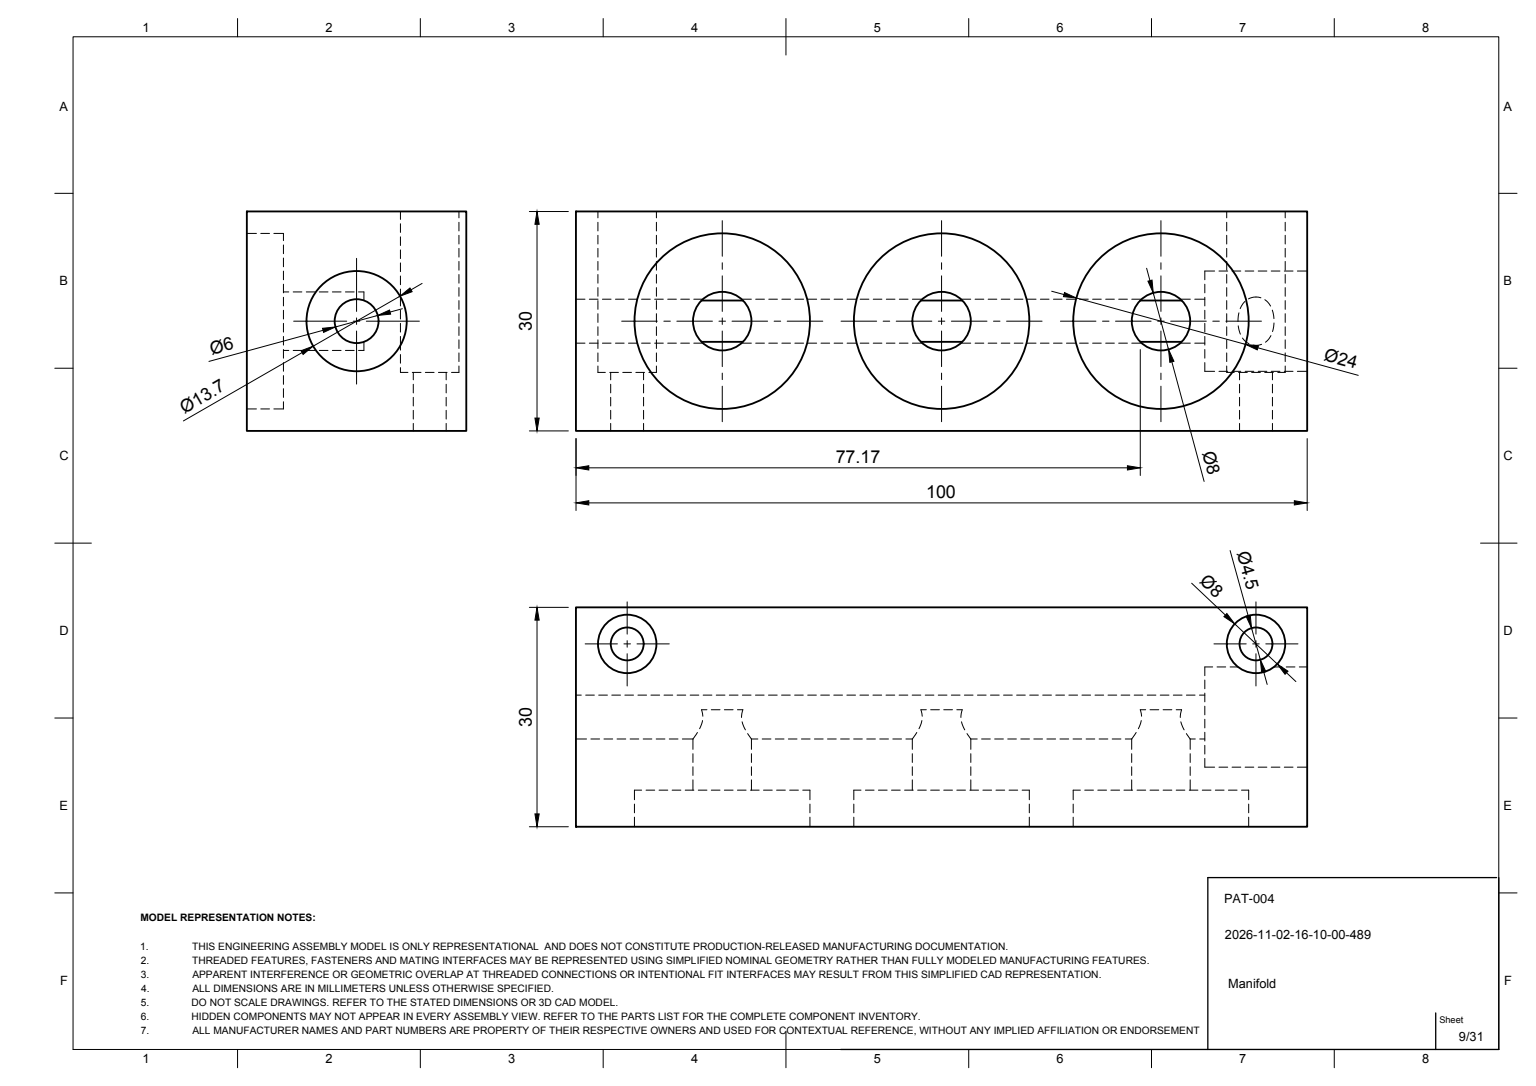
ISO-10303-21;
HEADER;
/* Generated by software containing ST-Developer
 * from STEP Tools, Inc. (www.steptools.com) 
 */

FILE_DESCRIPTION(
/* description */ ('Air blow-off nozzle station'),
/* implementation_level */ '2;1');

FILE_NAME(
/* name */ 'Manifold.step',
/* time_stamp */ '2026-10-27T10:53:54-07:00',
/* author */ (''),
/* organization */ (''),
/* preprocessor_version */ 'ST-DEVELOPER v20.2',
/* originating_system */ 'Autodesk Translation Framework v15.17.0.0',
/* authorisation */ '');

FILE_SCHEMA (('AUTOMOTIVE_DESIGN { 1 0 10303 214 3 1 1 }'));
ENDSEC;

DATA;
#10=MECHANICAL_DESIGN_GEOMETRIC_PRESENTATION_REPRESENTATION('',(#241),#7897);
#171=B_SPLINE_CURVE_WITH_KNOTS('',3,(#6538,#6539,#6540,#6541,#6542,#6543,
#6544,#6545,#6546,#6547,#6548,#6549),.UNSPECIFIED.,.F.,.F.,(4,2,2,2,2,4),
(-0.956775615070493,-0.896341583425285,-0.835907551780076,-0.715039488489658,
-0.596713648012452,-0.478387807535247),.UNSPECIFIED.);
#172=B_SPLINE_CURVE_WITH_KNOTS('',3,(#6550,#6551,#6552,#6553,#6554,#6555),
 .UNSPECIFIED.,.F.,.F.,(4,2,4),(-1.05899336181655,-1.0172096467157,-0.956775615070493),
 .UNSPECIFIED.);
#173=B_SPLINE_CURVE_WITH_KNOTS('',3,(#6557,#6558,#6559,#6560,#6561,#6562),
 .UNSPECIFIED.,.F.,.F.,(4,2,4),(0.956775615070494,1.0172096467157,1.0589933625076),
 .UNSPECIFIED.);
#174=B_SPLINE_CURVE_WITH_KNOTS('',3,(#6564,#6565,#6566,#6567,#6568,#6569,
#6570,#6571,#6572,#6573,#6574,#6575,#6576,#6577,#6578,#6579,#6580,#6581,
#6582,#6583,#6584,#6585,#6586,#6587,#6588,#6589,#6590),.UNSPECIFIED.,.F.,
 .F.,(4,2,3,2,2,2,2,2,2,2,2,2,4),(-0.102217746746059,-0.0604340316452088,
0.,0.0604340316452089,0.120868063290418,0.241736126580836,0.360061967058041,
0.478387807535247,0.596713648012453,0.715039488489658,0.835907551780076,
0.896341583425285,0.956775615070494),.UNSPECIFIED.);
#175=B_SPLINE_CURVE_WITH_KNOTS('',3,(#6593,#6594,#6595,#6596,#6597,#6598,
#6599,#6600,#6601,#6602,#6603,#6604,#6605,#6606,#6607,#6608,#6609),
 .UNSPECIFIED.,.F.,.F.,(4,2,2,2,2,3,2,4),(-0.478387807535247,-0.360061967058041,
-0.241736126580835,-0.120868063290418,-0.0604340316452086,2.22044604925031E-16,
0.0604340316452088,0.102217747437109),.UNSPECIFIED.);
#176=B_SPLINE_CURVE_WITH_KNOTS('',3,(#6630,#6631,#6632,#6633,#6634,#6635,
#6636,#6637,#6638,#6639,#6640,#6641),.UNSPECIFIED.,.F.,.F.,(4,2,2,2,2,4),
(-0.956775615070493,-0.896341583425285,-0.835907551780076,-0.715039488489658,
-0.596713648012452,-0.478387807535247),.UNSPECIFIED.);
#177=B_SPLINE_CURVE_WITH_KNOTS('',3,(#6642,#6643,#6644,#6645,#6646,#6647),
 .UNSPECIFIED.,.F.,.F.,(4,2,4),(-1.05899336181655,-1.0172096467157,-0.956775615070493),
 .UNSPECIFIED.);
#178=B_SPLINE_CURVE_WITH_KNOTS('',3,(#6649,#6650,#6651,#6652,#6653,#6654),
 .UNSPECIFIED.,.F.,.F.,(4,2,4),(0.956775615070493,1.0172096467157,1.0589933625076),
 .UNSPECIFIED.);
#179=B_SPLINE_CURVE_WITH_KNOTS('',3,(#6656,#6657,#6658,#6659,#6660,#6661,
#6662,#6663,#6664,#6665,#6666,#6667,#6668,#6669,#6670,#6671,#6672,#6673,
#6674,#6675,#6676,#6677,#6678,#6679,#6680,#6681,#6682),.UNSPECIFIED.,.F.,
 .F.,(4,2,3,2,2,2,2,2,2,2,2,2,4),(-0.102217746746057,-0.0604340316452088,
0.,0.0604340316452089,0.120868063290418,0.241736126580835,0.360061967058041,
0.478387807535247,0.596713648012452,0.715039488489658,0.835907551780075,
0.896341583425284,0.956775615070493),.UNSPECIFIED.);
#180=B_SPLINE_CURVE_WITH_KNOTS('',3,(#6685,#6686,#6687,#6688,#6689,#6690,
#6691,#6692,#6693,#6694,#6695,#6696,#6697,#6698,#6699,#6700,#6701),
 .UNSPECIFIED.,.F.,.F.,(4,2,2,2,2,3,2,4),(-0.478387807535247,-0.360061967058041,
-0.241736126580836,-0.120868063290418,-0.060434031645209,0.,0.0604340316452088,
0.102217747437111),.UNSPECIFIED.);
#181=B_SPLINE_CURVE_WITH_KNOTS('',3,(#6722,#6723,#6724,#6725,#6726,#6727,
#6728,#6729,#6730,#6731,#6732,#6733),.UNSPECIFIED.,.F.,.F.,(4,2,2,2,2,4),
(-0.956775615070493,-0.896341583425285,-0.835907551780076,-0.715039488489658,
-0.596713648012452,-0.478387807535247),.UNSPECIFIED.);
#182=B_SPLINE_CURVE_WITH_KNOTS('',3,(#6734,#6735,#6736,#6737,#6738,#6739),
 .UNSPECIFIED.,.F.,.F.,(4,2,4),(-1.05899336181655,-1.0172096467157,-0.956775615070493),
 .UNSPECIFIED.);
#183=B_SPLINE_CURVE_WITH_KNOTS('',3,(#6741,#6742,#6743,#6744,#6745,#6746),
 .UNSPECIFIED.,.F.,.F.,(4,2,4),(0.956775615070494,1.0172096467157,1.0589933625076),
 .UNSPECIFIED.);
#184=B_SPLINE_CURVE_WITH_KNOTS('',3,(#6748,#6749,#6750,#6751,#6752,#6753,
#6754,#6755,#6756,#6757,#6758,#6759,#6760,#6761,#6762,#6763,#6764,#6765,
#6766,#6767,#6768,#6769,#6770,#6771,#6772,#6773,#6774),.UNSPECIFIED.,.F.,
 .F.,(4,2,3,2,2,2,2,2,2,2,2,2,4),(-0.102217746746057,-0.0604340316452088,
0.,0.0604340316452089,0.120868063290418,0.241736126580836,0.360061967058041,
0.478387807535247,0.596713648012453,0.715039488489658,0.835907551780076,
0.896341583425285,0.956775615070494),.UNSPECIFIED.);
#185=B_SPLINE_CURVE_WITH_KNOTS('',3,(#6777,#6778,#6779,#6780,#6781,#6782,
#6783,#6784,#6785,#6786,#6787,#6788,#6789,#6790,#6791,#6792,#6793),
 .UNSPECIFIED.,.F.,.F.,(4,2,2,2,2,3,2,4),(-0.478387807535247,-0.360061967058041,
-0.241736126580835,-0.120868063290418,-0.0604340316452086,2.22044604925031E-16,
0.0604340316452088,0.102217747437111),.UNSPECIFIED.);
#186=B_SPLINE_CURVE_WITH_KNOTS('',3,(#6810,#6811,#6812,#6813,#6814,#6815,
#6816,#6817,#6818,#6819,#6820,#6821,#6822,#6823,#6824,#6825,#6826,#6827,
#6828,#6829,#6830,#6831,#6832,#6833,#6834,#6835,#6836,#6837,#6838,#6839,
#6840,#6841,#6842,#6843,#6844,#6845,#6846,#6847,#6848,#6849,#6850,#6851),
 .UNSPECIFIED.,.T.,.F.,(4,2,2,2,2,2,2,2,2,2,2,2,2,2,2,2,2,2,2,2,4),(0.,
0.0876674059984988,0.175334811996998,0.268557118055512,0.358098480537522,
0.447639843019532,0.537181205501541,0.626722567983551,0.719944874042066,
0.807612280040565,0.895279686039063,0.982947092037562,1.07061449803606,
1.16383680409458,1.25337816657659,1.3429195290586,1.43246089154061,1.52200225402261,
1.61522456008113,1.70289196607963,1.79055937207813),.UNSPECIFIED.);
#191=SHAPE_REPRESENTATION_RELATIONSHIP('SRR','None',#8005,#216);
#216=ADVANCED_BREP_SHAPE_REPRESENTATION('',(#266),#7872);
#241=STYLED_ITEM('',(#8234),#266);
#266=MANIFOLD_SOLID_BREP('Body1',#4290);
#293=FACE_BOUND('',#837,.T.);
#294=FACE_BOUND('',#843,.T.);
#295=FACE_BOUND('',#849,.T.);
#296=FACE_BOUND('',#851,.T.);
#297=FACE_BOUND('',#853,.T.);
#298=FACE_BOUND('',#857,.T.);
#299=FACE_BOUND('',#859,.T.);
#300=FACE_BOUND('',#861,.T.);
#301=FACE_BOUND('',#866,.T.);
#302=FACE_BOUND('',#868,.T.);
#303=FACE_BOUND('',#869,.T.);
#304=FACE_BOUND('',#870,.T.);
#305=FACE_BOUND('',#872,.T.);
#306=FACE_BOUND('',#874,.T.);
#307=FACE_BOUND('',#875,.T.);
#308=FACE_BOUND('',#877,.T.);
#309=FACE_BOUND('',#878,.T.);
#395=PLANE('',#4632);
#396=PLANE('',#4637);
#397=PLANE('',#4641);
#398=PLANE('',#4642);
#399=PLANE('',#4647);
#400=PLANE('',#4651);
#401=PLANE('',#4652);
#402=PLANE('',#4657);
#403=PLANE('',#4661);
#404=PLANE('',#4665);
#405=PLANE('',#4672);
#406=PLANE('',#4677);
#407=PLANE('',#4683);
#408=PLANE('',#4684);
#409=PLANE('',#4685);
#410=PLANE('',#4686);
#411=PLANE('',#4687);
#412=PLANE('',#4688);
#568=FACE_OUTER_BOUND('',#832,.T.);
#569=FACE_OUTER_BOUND('',#833,.T.);
#570=FACE_OUTER_BOUND('',#834,.T.);
#571=FACE_OUTER_BOUND('',#835,.T.);
#572=FACE_OUTER_BOUND('',#836,.T.);
#573=FACE_OUTER_BOUND('',#838,.T.);
#574=FACE_OUTER_BOUND('',#839,.T.);
#575=FACE_OUTER_BOUND('',#840,.T.);
#576=FACE_OUTER_BOUND('',#841,.T.);
#577=FACE_OUTER_BOUND('',#842,.T.);
#578=FACE_OUTER_BOUND('',#844,.T.);
#579=FACE_OUTER_BOUND('',#845,.T.);
#580=FACE_OUTER_BOUND('',#846,.T.);
#581=FACE_OUTER_BOUND('',#847,.T.);
#582=FACE_OUTER_BOUND('',#848,.T.);
#583=FACE_OUTER_BOUND('',#850,.T.);
#584=FACE_OUTER_BOUND('',#852,.T.);
#585=FACE_OUTER_BOUND('',#854,.T.);
#586=FACE_OUTER_BOUND('',#855,.T.);
#587=FACE_OUTER_BOUND('',#856,.T.);
#588=FACE_OUTER_BOUND('',#858,.T.);
#589=FACE_OUTER_BOUND('',#860,.T.);
#590=FACE_OUTER_BOUND('',#862,.T.);
#591=FACE_OUTER_BOUND('',#863,.T.);
#592=FACE_OUTER_BOUND('',#864,.T.);
#593=FACE_OUTER_BOUND('',#865,.T.);
#594=FACE_OUTER_BOUND('',#867,.T.);
#595=FACE_OUTER_BOUND('',#871,.T.);
#596=FACE_OUTER_BOUND('',#873,.T.);
#597=FACE_OUTER_BOUND('',#876,.T.);
#832=EDGE_LOOP('',(#3017,#3018));
#833=EDGE_LOOP('',(#3019,#3020,#3021,#3022,#3023,#3024,#3025,#3026,#3027,
#3028));
#834=EDGE_LOOP('',(#3029,#3030));
#835=EDGE_LOOP('',(#3031,#3032,#3033,#3034));
#836=EDGE_LOOP('',(#3035));
#837=EDGE_LOOP('',(#3036));
#838=EDGE_LOOP('',(#3037,#3038));
#839=EDGE_LOOP('',(#3039,#3040,#3041,#3042,#3043,#3044,#3045,#3046,#3047,
#3048));
#840=EDGE_LOOP('',(#3049,#3050));
#841=EDGE_LOOP('',(#3051,#3052,#3053,#3054));
#842=EDGE_LOOP('',(#3055));
#843=EDGE_LOOP('',(#3056));
#844=EDGE_LOOP('',(#3057,#3058));
#845=EDGE_LOOP('',(#3059,#3060,#3061,#3062,#3063,#3064,#3065,#3066,#3067,
#3068));
#846=EDGE_LOOP('',(#3069,#3070));
#847=EDGE_LOOP('',(#3071,#3072,#3073,#3074));
#848=EDGE_LOOP('',(#3075));
#849=EDGE_LOOP('',(#3076));
#850=EDGE_LOOP('',(#3077,#3078,#3079,#3080));
#851=EDGE_LOOP('',(#3081));
#852=EDGE_LOOP('',(#3082));
#853=EDGE_LOOP('',(#3083));
#854=EDGE_LOOP('',(#3084,#3085,#3086,#3087,#3088,#3089,#3090,#3091,#3092,
#3093,#3094,#3095,#3096,#3097,#3098,#3099,#3100,#3101,#3102,#3103,#3104,
#3105,#3106,#3107,#3108,#3109,#3110,#3111,#3112,#3113,#3114));
#855=EDGE_LOOP('',(#3115,#3116,#3117,#3118));
#856=EDGE_LOOP('',(#3119));
#857=EDGE_LOOP('',(#3120));
#858=EDGE_LOOP('',(#3121,#3122,#3123,#3124));
#859=EDGE_LOOP('',(#3125));
#860=EDGE_LOOP('',(#3126));
#861=EDGE_LOOP('',(#3127));
#862=EDGE_LOOP('',(#3128,#3129,#3130,#3131));
#863=EDGE_LOOP('',(#3132,#3133,#3134,#3135));
#864=EDGE_LOOP('',(#3136,#3137,#3138,#3139));
#865=EDGE_LOOP('',(#3140,#3141,#3142,#3143));
#866=EDGE_LOOP('',(#3144));
#867=EDGE_LOOP('',(#3145,#3146,#3147,#3148));
#868=EDGE_LOOP('',(#3149));
#869=EDGE_LOOP('',(#3150));
#870=EDGE_LOOP('',(#3151));
#871=EDGE_LOOP('',(#3152,#3153,#3154,#3155));
#872=EDGE_LOOP('',(#3156));
#873=EDGE_LOOP('',(#3157,#3158,#3159,#3160));
#874=EDGE_LOOP('',(#3161));
#875=EDGE_LOOP('',(#3162));
#876=EDGE_LOOP('',(#3163,#3164,#3165,#3166));
#877=EDGE_LOOP('',(#3167));
#878=EDGE_LOOP('',(#3168));
#1190=LINE('',#6530,#1544);
#1191=LINE('',#6536,#1545);
#1192=LINE('',#6611,#1546);
#1193=LINE('',#6616,#1547);
#1194=LINE('',#6622,#1548);
#1195=LINE('',#6628,#1549);
#1196=LINE('',#6703,#1550);
#1197=LINE('',#6708,#1551);
#1198=LINE('',#6714,#1552);
#1199=LINE('',#6720,#1553);
#1200=LINE('',#6795,#1554);
#1201=LINE('',#6800,#1555);
#1202=LINE('',#6807,#1556);
#1203=LINE('',#6858,#1557);
#1204=LINE('',#6859,#1558);
#1205=LINE('',#6860,#1559);
#1206=LINE('',#6861,#1560);
#1207=LINE('',#6866,#1561);
#1208=LINE('',#6875,#1562);
#1209=LINE('',#6883,#1563);
#1210=LINE('',#6887,#1564);
#1211=LINE('',#6891,#1565);
#1212=LINE('',#6893,#1566);
#1213=LINE('',#6895,#1567);
#1214=LINE('',#6896,#1568);
#1215=LINE('',#6899,#1569);
#1216=LINE('',#6901,#1570);
#1217=LINE('',#6902,#1571);
#1218=LINE('',#6905,#1572);
#1219=LINE('',#6907,#1573);
#1220=LINE('',#6908,#1574);
#1221=LINE('',#6910,#1575);
#1222=LINE('',#6911,#1576);
#1544=VECTOR('',#5212,1.);
#1545=VECTOR('',#5219,0.4);
#1546=VECTOR('',#5224,1.);
#1547=VECTOR('',#5229,1.2);
#1548=VECTOR('',#5236,1.);
#1549=VECTOR('',#5243,0.4);
#1550=VECTOR('',#5248,1.);
#1551=VECTOR('',#5253,1.2);
#1552=VECTOR('',#5260,1.);
#1553=VECTOR('',#5267,0.4);
#1554=VECTOR('',#5272,1.);
#1555=VECTOR('',#5277,1.2);
#1556=VECTOR('',#5286,0.684999999999999);
#1557=VECTOR('',#5297,0.300000000000001);
#1558=VECTOR('',#5298,0.300000000000001);
#1559=VECTOR('',#5299,0.300000000000001);
#1560=VECTOR('',#5300,0.300000000000001);
#1561=VECTOR('',#5305,0.4);
#1562=VECTOR('',#5316,0.4);
#1563=VECTOR('',#5327,0.225);
#1564=VECTOR('',#5332,0.225);
#1565=VECTOR('',#5335,1.);
#1566=VECTOR('',#5336,1.);
#1567=VECTOR('',#5337,1.);
#1568=VECTOR('',#5338,1.);
#1569=VECTOR('',#5341,1.);
#1570=VECTOR('',#5342,1.);
#1571=VECTOR('',#5343,1.);
#1572=VECTOR('',#5346,1.);
#1573=VECTOR('',#5347,1.);
#1574=VECTOR('',#5348,1.);
#1575=VECTOR('',#5351,1.);
#1576=VECTOR('',#5352,1.);
#1854=CIRCLE('',#4633,0.4);
#1855=CIRCLE('',#4635,0.4);
#1856=CIRCLE('',#4636,0.4);
#1857=CIRCLE('',#4639,1.2);
#1858=CIRCLE('',#4640,1.2);
#1859=CIRCLE('',#4643,0.4);
#1860=CIRCLE('',#4645,0.4);
#1861=CIRCLE('',#4646,0.4);
#1862=CIRCLE('',#4649,1.2);
#1863=CIRCLE('',#4650,1.2);
#1864=CIRCLE('',#4653,0.4);
#1865=CIRCLE('',#4655,0.4);
#1866=CIRCLE('',#4656,0.4);
#1867=CIRCLE('',#4659,1.2);
#1868=CIRCLE('',#4660,1.2);
#1869=CIRCLE('',#4663,0.684999999999999);
#1870=CIRCLE('',#4664,0.684999999999999);
#1871=CIRCLE('',#4666,0.300000000000001);
#1872=CIRCLE('',#4668,0.300000000000001);
#1873=CIRCLE('',#4670,0.4);
#1874=CIRCLE('',#4671,0.4);
#1875=CIRCLE('',#4673,0.225);
#1876=CIRCLE('',#4675,0.4);
#1877=CIRCLE('',#4676,0.4);
#1878=CIRCLE('',#4678,0.225);
#1879=CIRCLE('',#4680,0.225);
#1880=CIRCLE('',#4682,0.225);
#2047=VERTEX_POINT('',#6528);
#2048=VERTEX_POINT('',#6529);
#2049=VERTEX_POINT('',#6533);
#2050=VERTEX_POINT('',#6535);
#2051=VERTEX_POINT('',#6537);
#2052=VERTEX_POINT('',#6556);
#2053=VERTEX_POINT('',#6563);
#2054=VERTEX_POINT('',#6591);
#2055=VERTEX_POINT('',#6613);
#2056=VERTEX_POINT('',#6615);
#2057=VERTEX_POINT('',#6620);
#2058=VERTEX_POINT('',#6621);
#2059=VERTEX_POINT('',#6625);
#2060=VERTEX_POINT('',#6627);
#2061=VERTEX_POINT('',#6629);
#2062=VERTEX_POINT('',#6648);
#2063=VERTEX_POINT('',#6655);
#2064=VERTEX_POINT('',#6683);
#2065=VERTEX_POINT('',#6705);
#2066=VERTEX_POINT('',#6707);
#2067=VERTEX_POINT('',#6712);
#2068=VERTEX_POINT('',#6713);
#2069=VERTEX_POINT('',#6717);
#2070=VERTEX_POINT('',#6719);
#2071=VERTEX_POINT('',#6721);
#2072=VERTEX_POINT('',#6740);
#2073=VERTEX_POINT('',#6747);
#2074=VERTEX_POINT('',#6775);
#2075=VERTEX_POINT('',#6797);
#2076=VERTEX_POINT('',#6799);
#2077=VERTEX_POINT('',#6804);
#2078=VERTEX_POINT('',#6806);
#2079=VERTEX_POINT('',#6809);
#2080=VERTEX_POINT('',#6853);
#2081=VERTEX_POINT('',#6856);
#2082=VERTEX_POINT('',#6863);
#2083=VERTEX_POINT('',#6865);
#2084=VERTEX_POINT('',#6869);
#2085=VERTEX_POINT('',#6872);
#2086=VERTEX_POINT('',#6874);
#2087=VERTEX_POINT('',#6878);
#2088=VERTEX_POINT('',#6881);
#2089=VERTEX_POINT('',#6885);
#2090=VERTEX_POINT('',#6889);
#2091=VERTEX_POINT('',#6890);
#2092=VERTEX_POINT('',#6892);
#2093=VERTEX_POINT('',#6894);
#2094=VERTEX_POINT('',#6898);
#2095=VERTEX_POINT('',#6900);
#2096=VERTEX_POINT('',#6904);
#2097=VERTEX_POINT('',#6906);
#2426=EDGE_CURVE('',#2047,#2048,#1190,.T.);
#2427=EDGE_CURVE('',#2048,#2047,#1854,.T.);
#2428=EDGE_CURVE('',#2049,#2049,#1855,.T.);
#2429=EDGE_CURVE('',#2049,#2050,#1191,.T.);
#2430=EDGE_CURVE('',#2051,#2050,#171,.T.);
#2431=EDGE_CURVE('',#2048,#2051,#172,.T.);
#2432=EDGE_CURVE('',#2052,#2047,#173,.T.);
#2433=EDGE_CURVE('',#2053,#2052,#174,.T.);
#2434=EDGE_CURVE('',#2053,#2054,#1856,.T.);
#2435=EDGE_CURVE('',#2050,#2054,#175,.T.);
#2436=EDGE_CURVE('',#2054,#2053,#1192,.T.);
#2437=EDGE_CURVE('',#2055,#2055,#1857,.T.);
#2438=EDGE_CURVE('',#2055,#2056,#1193,.T.);
#2439=EDGE_CURVE('',#2056,#2056,#1858,.T.);
#2440=EDGE_CURVE('',#2057,#2058,#1194,.T.);
#2441=EDGE_CURVE('',#2058,#2057,#1859,.T.);
#2442=EDGE_CURVE('',#2059,#2059,#1860,.T.);
#2443=EDGE_CURVE('',#2059,#2060,#1195,.T.);
#2444=EDGE_CURVE('',#2061,#2060,#176,.T.);
#2445=EDGE_CURVE('',#2058,#2061,#177,.T.);
#2446=EDGE_CURVE('',#2062,#2057,#178,.T.);
#2447=EDGE_CURVE('',#2063,#2062,#179,.T.);
#2448=EDGE_CURVE('',#2063,#2064,#1861,.T.);
#2449=EDGE_CURVE('',#2060,#2064,#180,.T.);
#2450=EDGE_CURVE('',#2064,#2063,#1196,.T.);
#2451=EDGE_CURVE('',#2065,#2065,#1862,.T.);
#2452=EDGE_CURVE('',#2065,#2066,#1197,.T.);
#2453=EDGE_CURVE('',#2066,#2066,#1863,.T.);
#2454=EDGE_CURVE('',#2067,#2068,#1198,.T.);
#2455=EDGE_CURVE('',#2068,#2067,#1864,.T.);
#2456=EDGE_CURVE('',#2069,#2069,#1865,.T.);
#2457=EDGE_CURVE('',#2069,#2070,#1199,.T.);
#2458=EDGE_CURVE('',#2071,#2070,#181,.T.);
#2459=EDGE_CURVE('',#2068,#2071,#182,.T.);
#2460=EDGE_CURVE('',#2072,#2067,#183,.T.);
#2461=EDGE_CURVE('',#2073,#2072,#184,.T.);
#2462=EDGE_CURVE('',#2073,#2074,#1866,.T.);
#2463=EDGE_CURVE('',#2070,#2074,#185,.T.);
#2464=EDGE_CURVE('',#2074,#2073,#1200,.T.);
#2465=EDGE_CURVE('',#2075,#2075,#1867,.T.);
#2466=EDGE_CURVE('',#2075,#2076,#1201,.T.);
#2467=EDGE_CURVE('',#2076,#2076,#1868,.T.);
#2468=EDGE_CURVE('',#2077,#2077,#1869,.T.);
#2469=EDGE_CURVE('',#2077,#2078,#1202,.T.);
#2470=EDGE_CURVE('',#2078,#2078,#1870,.T.);
#2471=EDGE_CURVE('',#2079,#2079,#186,.T.);
#2472=EDGE_CURVE('',#2080,#2080,#1871,.T.);
#2473=EDGE_CURVE('',#2081,#2081,#1872,.T.);
#2474=EDGE_CURVE('',#2081,#2071,#1203,.T.);
#2475=EDGE_CURVE('',#2072,#2061,#1204,.T.);
#2476=EDGE_CURVE('',#2062,#2051,#1205,.T.);
#2477=EDGE_CURVE('',#2052,#2080,#1206,.T.);
#2478=EDGE_CURVE('',#2082,#2082,#1873,.T.);
#2479=EDGE_CURVE('',#2082,#2083,#1207,.T.);
#2480=EDGE_CURVE('',#2083,#2083,#1874,.T.);
#2481=EDGE_CURVE('',#2084,#2084,#1875,.T.);
#2482=EDGE_CURVE('',#2085,#2085,#1876,.T.);
#2483=EDGE_CURVE('',#2085,#2086,#1208,.T.);
#2484=EDGE_CURVE('',#2086,#2086,#1877,.T.);
#2485=EDGE_CURVE('',#2087,#2087,#1878,.T.);
#2486=EDGE_CURVE('',#2088,#2088,#1879,.T.);
#2487=EDGE_CURVE('',#2088,#2084,#1209,.T.);
#2488=EDGE_CURVE('',#2089,#2089,#1880,.T.);
#2489=EDGE_CURVE('',#2089,#2087,#1210,.T.);
#2490=EDGE_CURVE('',#2090,#2091,#1211,.T.);
#2491=EDGE_CURVE('',#2091,#2092,#1212,.T.);
#2492=EDGE_CURVE('',#2093,#2092,#1213,.T.);
#2493=EDGE_CURVE('',#2090,#2093,#1214,.T.);
#2494=EDGE_CURVE('',#2094,#2090,#1215,.T.);
#2495=EDGE_CURVE('',#2095,#2093,#1216,.T.);
#2496=EDGE_CURVE('',#2094,#2095,#1217,.T.);
#2497=EDGE_CURVE('',#2096,#2094,#1218,.T.);
#2498=EDGE_CURVE('',#2097,#2095,#1219,.T.);
#2499=EDGE_CURVE('',#2096,#2097,#1220,.T.);
#2500=EDGE_CURVE('',#2091,#2096,#1221,.T.);
#2501=EDGE_CURVE('',#2092,#2097,#1222,.T.);
#3017=ORIENTED_EDGE('',*,*,#2426,.F.);
#3018=ORIENTED_EDGE('',*,*,#2427,.F.);
#3019=ORIENTED_EDGE('',*,*,#2428,.F.);
#3020=ORIENTED_EDGE('',*,*,#2429,.T.);
#3021=ORIENTED_EDGE('',*,*,#2430,.F.);
#3022=ORIENTED_EDGE('',*,*,#2431,.F.);
#3023=ORIENTED_EDGE('',*,*,#2427,.T.);
#3024=ORIENTED_EDGE('',*,*,#2432,.F.);
#3025=ORIENTED_EDGE('',*,*,#2433,.F.);
#3026=ORIENTED_EDGE('',*,*,#2434,.T.);
#3027=ORIENTED_EDGE('',*,*,#2435,.F.);
#3028=ORIENTED_EDGE('',*,*,#2429,.F.);
#3029=ORIENTED_EDGE('',*,*,#2436,.F.);
#3030=ORIENTED_EDGE('',*,*,#2434,.F.);
#3031=ORIENTED_EDGE('',*,*,#2437,.F.);
#3032=ORIENTED_EDGE('',*,*,#2438,.T.);
#3033=ORIENTED_EDGE('',*,*,#2439,.T.);
#3034=ORIENTED_EDGE('',*,*,#2438,.F.);
#3035=ORIENTED_EDGE('',*,*,#2439,.F.);
#3036=ORIENTED_EDGE('',*,*,#2428,.T.);
#3037=ORIENTED_EDGE('',*,*,#2440,.F.);
#3038=ORIENTED_EDGE('',*,*,#2441,.F.);
#3039=ORIENTED_EDGE('',*,*,#2442,.F.);
#3040=ORIENTED_EDGE('',*,*,#2443,.T.);
#3041=ORIENTED_EDGE('',*,*,#2444,.F.);
#3042=ORIENTED_EDGE('',*,*,#2445,.F.);
#3043=ORIENTED_EDGE('',*,*,#2441,.T.);
#3044=ORIENTED_EDGE('',*,*,#2446,.F.);
#3045=ORIENTED_EDGE('',*,*,#2447,.F.);
#3046=ORIENTED_EDGE('',*,*,#2448,.T.);
#3047=ORIENTED_EDGE('',*,*,#2449,.F.);
#3048=ORIENTED_EDGE('',*,*,#2443,.F.);
#3049=ORIENTED_EDGE('',*,*,#2450,.F.);
#3050=ORIENTED_EDGE('',*,*,#2448,.F.);
#3051=ORIENTED_EDGE('',*,*,#2451,.F.);
#3052=ORIENTED_EDGE('',*,*,#2452,.T.);
#3053=ORIENTED_EDGE('',*,*,#2453,.T.);
#3054=ORIENTED_EDGE('',*,*,#2452,.F.);
#3055=ORIENTED_EDGE('',*,*,#2453,.F.);
#3056=ORIENTED_EDGE('',*,*,#2442,.T.);
#3057=ORIENTED_EDGE('',*,*,#2454,.F.);
#3058=ORIENTED_EDGE('',*,*,#2455,.F.);
#3059=ORIENTED_EDGE('',*,*,#2456,.F.);
#3060=ORIENTED_EDGE('',*,*,#2457,.T.);
#3061=ORIENTED_EDGE('',*,*,#2458,.F.);
#3062=ORIENTED_EDGE('',*,*,#2459,.F.);
#3063=ORIENTED_EDGE('',*,*,#2455,.T.);
#3064=ORIENTED_EDGE('',*,*,#2460,.F.);
#3065=ORIENTED_EDGE('',*,*,#2461,.F.);
#3066=ORIENTED_EDGE('',*,*,#2462,.T.);
#3067=ORIENTED_EDGE('',*,*,#2463,.F.);
#3068=ORIENTED_EDGE('',*,*,#2457,.F.);
#3069=ORIENTED_EDGE('',*,*,#2464,.F.);
#3070=ORIENTED_EDGE('',*,*,#2462,.F.);
#3071=ORIENTED_EDGE('',*,*,#2465,.F.);
#3072=ORIENTED_EDGE('',*,*,#2466,.T.);
#3073=ORIENTED_EDGE('',*,*,#2467,.T.);
#3074=ORIENTED_EDGE('',*,*,#2466,.F.);
#3075=ORIENTED_EDGE('',*,*,#2467,.F.);
#3076=ORIENTED_EDGE('',*,*,#2456,.T.);
#3077=ORIENTED_EDGE('',*,*,#2468,.F.);
#3078=ORIENTED_EDGE('',*,*,#2469,.T.);
#3079=ORIENTED_EDGE('',*,*,#2470,.F.);
#3080=ORIENTED_EDGE('',*,*,#2469,.F.);
#3081=ORIENTED_EDGE('',*,*,#2471,.F.);
#3082=ORIENTED_EDGE('',*,*,#2468,.T.);
#3083=ORIENTED_EDGE('',*,*,#2472,.F.);
#3084=ORIENTED_EDGE('',*,*,#2473,.F.);
#3085=ORIENTED_EDGE('',*,*,#2474,.T.);
#3086=ORIENTED_EDGE('',*,*,#2458,.T.);
#3087=ORIENTED_EDGE('',*,*,#2463,.T.);
#3088=ORIENTED_EDGE('',*,*,#2464,.T.);
#3089=ORIENTED_EDGE('',*,*,#2461,.T.);
#3090=ORIENTED_EDGE('',*,*,#2475,.T.);
#3091=ORIENTED_EDGE('',*,*,#2444,.T.);
#3092=ORIENTED_EDGE('',*,*,#2449,.T.);
#3093=ORIENTED_EDGE('',*,*,#2450,.T.);
#3094=ORIENTED_EDGE('',*,*,#2447,.T.);
#3095=ORIENTED_EDGE('',*,*,#2476,.T.);
#3096=ORIENTED_EDGE('',*,*,#2430,.T.);
#3097=ORIENTED_EDGE('',*,*,#2435,.T.);
#3098=ORIENTED_EDGE('',*,*,#2436,.T.);
#3099=ORIENTED_EDGE('',*,*,#2433,.T.);
#3100=ORIENTED_EDGE('',*,*,#2477,.T.);
#3101=ORIENTED_EDGE('',*,*,#2472,.T.);
#3102=ORIENTED_EDGE('',*,*,#2477,.F.);
#3103=ORIENTED_EDGE('',*,*,#2432,.T.);
#3104=ORIENTED_EDGE('',*,*,#2426,.T.);
#3105=ORIENTED_EDGE('',*,*,#2431,.T.);
#3106=ORIENTED_EDGE('',*,*,#2476,.F.);
#3107=ORIENTED_EDGE('',*,*,#2446,.T.);
#3108=ORIENTED_EDGE('',*,*,#2440,.T.);
#3109=ORIENTED_EDGE('',*,*,#2445,.T.);
#3110=ORIENTED_EDGE('',*,*,#2475,.F.);
#3111=ORIENTED_EDGE('',*,*,#2460,.T.);
#3112=ORIENTED_EDGE('',*,*,#2454,.T.);
#3113=ORIENTED_EDGE('',*,*,#2459,.T.);
#3114=ORIENTED_EDGE('',*,*,#2474,.F.);
#3115=ORIENTED_EDGE('',*,*,#2478,.F.);
#3116=ORIENTED_EDGE('',*,*,#2479,.T.);
#3117=ORIENTED_EDGE('',*,*,#2480,.F.);
#3118=ORIENTED_EDGE('',*,*,#2479,.F.);
#3119=ORIENTED_EDGE('',*,*,#2478,.T.);
#3120=ORIENTED_EDGE('',*,*,#2481,.F.);
#3121=ORIENTED_EDGE('',*,*,#2482,.F.);
#3122=ORIENTED_EDGE('',*,*,#2483,.T.);
#3123=ORIENTED_EDGE('',*,*,#2484,.F.);
#3124=ORIENTED_EDGE('',*,*,#2483,.F.);
#3125=ORIENTED_EDGE('',*,*,#2471,.T.);
#3126=ORIENTED_EDGE('',*,*,#2482,.T.);
#3127=ORIENTED_EDGE('',*,*,#2485,.F.);
#3128=ORIENTED_EDGE('',*,*,#2486,.F.);
#3129=ORIENTED_EDGE('',*,*,#2487,.T.);
#3130=ORIENTED_EDGE('',*,*,#2481,.T.);
#3131=ORIENTED_EDGE('',*,*,#2487,.F.);
#3132=ORIENTED_EDGE('',*,*,#2488,.F.);
#3133=ORIENTED_EDGE('',*,*,#2489,.T.);
#3134=ORIENTED_EDGE('',*,*,#2485,.T.);
#3135=ORIENTED_EDGE('',*,*,#2489,.F.);
#3136=ORIENTED_EDGE('',*,*,#2490,.T.);
#3137=ORIENTED_EDGE('',*,*,#2491,.T.);
#3138=ORIENTED_EDGE('',*,*,#2492,.F.);
#3139=ORIENTED_EDGE('',*,*,#2493,.F.);
#3140=ORIENTED_EDGE('',*,*,#2494,.T.);
#3141=ORIENTED_EDGE('',*,*,#2493,.T.);
#3142=ORIENTED_EDGE('',*,*,#2495,.F.);
#3143=ORIENTED_EDGE('',*,*,#2496,.F.);
#3144=ORIENTED_EDGE('',*,*,#2470,.T.);
#3145=ORIENTED_EDGE('',*,*,#2497,.T.);
#3146=ORIENTED_EDGE('',*,*,#2496,.T.);
#3147=ORIENTED_EDGE('',*,*,#2498,.F.);
#3148=ORIENTED_EDGE('',*,*,#2499,.F.);
#3149=ORIENTED_EDGE('',*,*,#2437,.T.);
#3150=ORIENTED_EDGE('',*,*,#2451,.T.);
#3151=ORIENTED_EDGE('',*,*,#2465,.T.);
#3152=ORIENTED_EDGE('',*,*,#2500,.T.);
#3153=ORIENTED_EDGE('',*,*,#2499,.T.);
#3154=ORIENTED_EDGE('',*,*,#2501,.F.);
#3155=ORIENTED_EDGE('',*,*,#2491,.F.);
#3156=ORIENTED_EDGE('',*,*,#2473,.T.);
#3157=ORIENTED_EDGE('',*,*,#2501,.T.);
#3158=ORIENTED_EDGE('',*,*,#2498,.T.);
#3159=ORIENTED_EDGE('',*,*,#2495,.T.);
#3160=ORIENTED_EDGE('',*,*,#2492,.T.);
#3161=ORIENTED_EDGE('',*,*,#2480,.T.);
#3162=ORIENTED_EDGE('',*,*,#2484,.T.);
#3163=ORIENTED_EDGE('',*,*,#2500,.F.);
#3164=ORIENTED_EDGE('',*,*,#2490,.F.);
#3165=ORIENTED_EDGE('',*,*,#2494,.F.);
#3166=ORIENTED_EDGE('',*,*,#2497,.F.);
#3167=ORIENTED_EDGE('',*,*,#2486,.T.);
#3168=ORIENTED_EDGE('',*,*,#2488,.T.);
#3963=CYLINDRICAL_SURFACE('',#4634,0.4);
#3964=CYLINDRICAL_SURFACE('',#4638,1.2);
#3965=CYLINDRICAL_SURFACE('',#4644,0.4);
#3966=CYLINDRICAL_SURFACE('',#4648,1.2);
#3967=CYLINDRICAL_SURFACE('',#4654,0.4);
#3968=CYLINDRICAL_SURFACE('',#4658,1.2);
#3969=CYLINDRICAL_SURFACE('',#4662,0.684999999999999);
#3970=CYLINDRICAL_SURFACE('',#4667,0.300000000000001);
#3971=CYLINDRICAL_SURFACE('',#4669,0.4);
#3972=CYLINDRICAL_SURFACE('',#4674,0.4);
#3973=CYLINDRICAL_SURFACE('',#4679,0.225);
#3974=CYLINDRICAL_SURFACE('',#4681,0.225);
#4058=ADVANCED_FACE('',(#568),#395,.F.);
#4059=ADVANCED_FACE('',(#569),#3963,.F.);
#4060=ADVANCED_FACE('',(#570),#396,.F.);
#4061=ADVANCED_FACE('',(#571),#3964,.F.);
#4062=ADVANCED_FACE('',(#572,#293),#397,.F.);
#4063=ADVANCED_FACE('',(#573),#398,.F.);
#4064=ADVANCED_FACE('',(#574),#3965,.F.);
#4065=ADVANCED_FACE('',(#575),#399,.F.);
#4066=ADVANCED_FACE('',(#576),#3966,.F.);
#4067=ADVANCED_FACE('',(#577,#294),#400,.F.);
#4068=ADVANCED_FACE('',(#578),#401,.F.);
#4069=ADVANCED_FACE('',(#579),#3967,.F.);
#4070=ADVANCED_FACE('',(#580),#402,.F.);
#4071=ADVANCED_FACE('',(#581),#3968,.F.);
#4072=ADVANCED_FACE('',(#582,#295),#403,.F.);
#4073=ADVANCED_FACE('',(#583,#296),#3969,.F.);
#4074=ADVANCED_FACE('',(#584,#297),#404,.T.);
#4075=ADVANCED_FACE('',(#585),#3970,.F.);
#4076=ADVANCED_FACE('',(#586),#3971,.F.);
#4077=ADVANCED_FACE('',(#587,#298),#405,.T.);
#4078=ADVANCED_FACE('',(#588,#299),#3972,.F.);
#4079=ADVANCED_FACE('',(#589,#300),#406,.T.);
#4080=ADVANCED_FACE('',(#590),#3973,.F.);
#4081=ADVANCED_FACE('',(#591),#3974,.F.);
#4082=ADVANCED_FACE('',(#592),#407,.T.);
#4083=ADVANCED_FACE('',(#593,#301),#408,.T.);
#4084=ADVANCED_FACE('',(#594,#302,#303,#304),#409,.T.);
#4085=ADVANCED_FACE('',(#595,#305),#410,.T.);
#4086=ADVANCED_FACE('',(#596,#306,#307),#411,.T.);
#4087=ADVANCED_FACE('',(#597,#308,#309),#412,.F.);
#4290=CLOSED_SHELL('',(#4058,#4059,#4060,#4061,#4062,#4063,#4064,#4065,
#4066,#4067,#4068,#4069,#4070,#4071,#4072,#4073,#4074,#4075,#4076,#4077,
#4078,#4079,#4080,#4081,#4082,#4083,#4084,#4085,#4086,#4087));
#4631=AXIS2_PLACEMENT_3D('',#6526,#5208,#5209);
#4632=AXIS2_PLACEMENT_3D('',#6527,#5210,#5211);
#4633=AXIS2_PLACEMENT_3D('',#6531,#5213,#5214);
#4634=AXIS2_PLACEMENT_3D('',#6532,#5215,#5216);
#4635=AXIS2_PLACEMENT_3D('',#6534,#5217,#5218);
#4636=AXIS2_PLACEMENT_3D('',#6592,#5220,#5221);
#4637=AXIS2_PLACEMENT_3D('',#6610,#5222,#5223);
#4638=AXIS2_PLACEMENT_3D('',#6612,#5225,#5226);
#4639=AXIS2_PLACEMENT_3D('',#6614,#5227,#5228);
#4640=AXIS2_PLACEMENT_3D('',#6617,#5230,#5231);
#4641=AXIS2_PLACEMENT_3D('',#6618,#5232,#5233);
#4642=AXIS2_PLACEMENT_3D('',#6619,#5234,#5235);
#4643=AXIS2_PLACEMENT_3D('',#6623,#5237,#5238);
#4644=AXIS2_PLACEMENT_3D('',#6624,#5239,#5240);
#4645=AXIS2_PLACEMENT_3D('',#6626,#5241,#5242);
#4646=AXIS2_PLACEMENT_3D('',#6684,#5244,#5245);
#4647=AXIS2_PLACEMENT_3D('',#6702,#5246,#5247);
#4648=AXIS2_PLACEMENT_3D('',#6704,#5249,#5250);
#4649=AXIS2_PLACEMENT_3D('',#6706,#5251,#5252);
#4650=AXIS2_PLACEMENT_3D('',#6709,#5254,#5255);
#4651=AXIS2_PLACEMENT_3D('',#6710,#5256,#5257);
#4652=AXIS2_PLACEMENT_3D('',#6711,#5258,#5259);
#4653=AXIS2_PLACEMENT_3D('',#6715,#5261,#5262);
#4654=AXIS2_PLACEMENT_3D('',#6716,#5263,#5264);
#4655=AXIS2_PLACEMENT_3D('',#6718,#5265,#5266);
#4656=AXIS2_PLACEMENT_3D('',#6776,#5268,#5269);
#4657=AXIS2_PLACEMENT_3D('',#6794,#5270,#5271);
#4658=AXIS2_PLACEMENT_3D('',#6796,#5273,#5274);
#4659=AXIS2_PLACEMENT_3D('',#6798,#5275,#5276);
#4660=AXIS2_PLACEMENT_3D('',#6801,#5278,#5279);
#4661=AXIS2_PLACEMENT_3D('',#6802,#5280,#5281);
#4662=AXIS2_PLACEMENT_3D('',#6803,#5282,#5283);
#4663=AXIS2_PLACEMENT_3D('',#6805,#5284,#5285);
#4664=AXIS2_PLACEMENT_3D('',#6808,#5287,#5288);
#4665=AXIS2_PLACEMENT_3D('',#6852,#5289,#5290);
#4666=AXIS2_PLACEMENT_3D('',#6854,#5291,#5292);
#4667=AXIS2_PLACEMENT_3D('',#6855,#5293,#5294);
#4668=AXIS2_PLACEMENT_3D('',#6857,#5295,#5296);
#4669=AXIS2_PLACEMENT_3D('',#6862,#5301,#5302);
#4670=AXIS2_PLACEMENT_3D('',#6864,#5303,#5304);
#4671=AXIS2_PLACEMENT_3D('',#6867,#5306,#5307);
#4672=AXIS2_PLACEMENT_3D('',#6868,#5308,#5309);
#4673=AXIS2_PLACEMENT_3D('',#6870,#5310,#5311);
#4674=AXIS2_PLACEMENT_3D('',#6871,#5312,#5313);
#4675=AXIS2_PLACEMENT_3D('',#6873,#5314,#5315);
#4676=AXIS2_PLACEMENT_3D('',#6876,#5317,#5318);
#4677=AXIS2_PLACEMENT_3D('',#6877,#5319,#5320);
#4678=AXIS2_PLACEMENT_3D('',#6879,#5321,#5322);
#4679=AXIS2_PLACEMENT_3D('',#6880,#5323,#5324);
#4680=AXIS2_PLACEMENT_3D('',#6882,#5325,#5326);
#4681=AXIS2_PLACEMENT_3D('',#6884,#5328,#5329);
#4682=AXIS2_PLACEMENT_3D('',#6886,#5330,#5331);
#4683=AXIS2_PLACEMENT_3D('',#6888,#5333,#5334);
#4684=AXIS2_PLACEMENT_3D('',#6897,#5339,#5340);
#4685=AXIS2_PLACEMENT_3D('',#6903,#5344,#5345);
#4686=AXIS2_PLACEMENT_3D('',#6909,#5349,#5350);
#4687=AXIS2_PLACEMENT_3D('',#6912,#5353,#5354);
#4688=AXIS2_PLACEMENT_3D('',#6913,#5355,#5356);
#5208=DIRECTION('axis',(0.,0.,1.));
#5209=DIRECTION('refdir',(1.,0.,0.));
#5210=DIRECTION('center_axis',(0.,1.,0.));
#5211=DIRECTION('ref_axis',(1.,0.,0.));
#5212=DIRECTION('',(-1.,0.,0.));
#5213=DIRECTION('center_axis',(0.,1.,0.));
#5214=DIRECTION('ref_axis',(1.,0.,0.));
#5215=DIRECTION('center_axis',(0.,1.,0.));
#5216=DIRECTION('ref_axis',(1.,0.,0.));
#5217=DIRECTION('center_axis',(0.,1.,0.));
#5218=DIRECTION('ref_axis',(1.,0.,0.));
#5219=DIRECTION('',(0.,1.,0.));
#5220=DIRECTION('center_axis',(0.,1.,0.));
#5221=DIRECTION('ref_axis',(1.,0.,0.));
#5222=DIRECTION('center_axis',(0.,1.,0.));
#5223=DIRECTION('ref_axis',(1.,0.,0.));
#5224=DIRECTION('',(1.,0.,0.));
#5225=DIRECTION('center_axis',(0.,1.,0.));
#5226=DIRECTION('ref_axis',(1.,0.,0.));
#5227=DIRECTION('center_axis',(0.,1.,0.));
#5228=DIRECTION('ref_axis',(1.,0.,0.));
#5229=DIRECTION('',(0.,1.,0.));
#5230=DIRECTION('center_axis',(0.,1.,0.));
#5231=DIRECTION('ref_axis',(1.,0.,0.));
#5232=DIRECTION('center_axis',(0.,1.,0.));
#5233=DIRECTION('ref_axis',(1.,0.,0.));
#5234=DIRECTION('center_axis',(0.,1.,0.));
#5235=DIRECTION('ref_axis',(1.,0.,0.));
#5236=DIRECTION('',(-1.,0.,0.));
#5237=DIRECTION('center_axis',(0.,1.,0.));
#5238=DIRECTION('ref_axis',(1.,0.,0.));
#5239=DIRECTION('center_axis',(0.,1.,0.));
#5240=DIRECTION('ref_axis',(1.,0.,0.));
#5241=DIRECTION('center_axis',(0.,1.,0.));
#5242=DIRECTION('ref_axis',(1.,0.,0.));
#5243=DIRECTION('',(0.,1.,0.));
#5244=DIRECTION('center_axis',(0.,1.,0.));
#5245=DIRECTION('ref_axis',(1.,0.,0.));
#5246=DIRECTION('center_axis',(0.,1.,0.));
#5247=DIRECTION('ref_axis',(1.,0.,0.));
#5248=DIRECTION('',(1.,0.,0.));
#5249=DIRECTION('center_axis',(0.,1.,0.));
#5250=DIRECTION('ref_axis',(1.,0.,0.));
#5251=DIRECTION('center_axis',(0.,1.,0.));
#5252=DIRECTION('ref_axis',(1.,0.,0.));
#5253=DIRECTION('',(0.,1.,0.));
#5254=DIRECTION('center_axis',(0.,1.,0.));
#5255=DIRECTION('ref_axis',(1.,0.,0.));
#5256=DIRECTION('center_axis',(0.,1.,0.));
#5257=DIRECTION('ref_axis',(1.,0.,0.));
#5258=DIRECTION('center_axis',(0.,1.,0.));
#5259=DIRECTION('ref_axis',(1.,0.,0.));
#5260=DIRECTION('',(-1.,0.,0.));
#5261=DIRECTION('center_axis',(0.,1.,0.));
#5262=DIRECTION('ref_axis',(1.,0.,0.));
#5263=DIRECTION('center_axis',(0.,1.,0.));
#5264=DIRECTION('ref_axis',(1.,0.,0.));
#5265=DIRECTION('center_axis',(0.,1.,0.));
#5266=DIRECTION('ref_axis',(1.,0.,0.));
#5267=DIRECTION('',(0.,1.,0.));
#5268=DIRECTION('center_axis',(0.,1.,0.));
#5269=DIRECTION('ref_axis',(1.,0.,0.));
#5270=DIRECTION('center_axis',(0.,1.,0.));
#5271=DIRECTION('ref_axis',(1.,0.,0.));
#5272=DIRECTION('',(1.,0.,0.));
#5273=DIRECTION('center_axis',(0.,1.,0.));
#5274=DIRECTION('ref_axis',(1.,0.,0.));
#5275=DIRECTION('center_axis',(0.,1.,0.));
#5276=DIRECTION('ref_axis',(1.,0.,0.));
#5277=DIRECTION('',(0.,1.,0.));
#5278=DIRECTION('center_axis',(0.,1.,0.));
#5279=DIRECTION('ref_axis',(1.,0.,0.));
#5280=DIRECTION('center_axis',(0.,1.,0.));
#5281=DIRECTION('ref_axis',(1.,0.,0.));
#5282=DIRECTION('center_axis',(1.,0.,0.));
#5283=DIRECTION('ref_axis',(0.,0.,-1.));
#5284=DIRECTION('center_axis',(1.,0.,0.));
#5285=DIRECTION('ref_axis',(0.,0.,-1.));
#5286=DIRECTION('',(1.,0.,0.));
#5287=DIRECTION('center_axis',(-1.,0.,0.));
#5288=DIRECTION('ref_axis',(0.,0.,-1.));
#5289=DIRECTION('center_axis',(1.,0.,0.));
#5290=DIRECTION('ref_axis',(0.,0.,-1.));
#5291=DIRECTION('center_axis',(1.,0.,0.));
#5292=DIRECTION('ref_axis',(0.,0.,-1.));
#5293=DIRECTION('center_axis',(1.,0.,0.));
#5294=DIRECTION('ref_axis',(0.,0.,-1.));
#5295=DIRECTION('center_axis',(1.,0.,0.));
#5296=DIRECTION('ref_axis',(0.,0.,-1.));
#5297=DIRECTION('',(1.,0.,0.));
#5298=DIRECTION('',(1.,0.,0.));
#5299=DIRECTION('',(1.,0.,0.));
#5300=DIRECTION('',(1.,0.,0.));
#5301=DIRECTION('center_axis',(0.,0.,1.));
#5302=DIRECTION('ref_axis',(1.,0.,0.));
#5303=DIRECTION('center_axis',(0.,0.,1.));
#5304=DIRECTION('ref_axis',(1.,0.,0.));
#5305=DIRECTION('',(0.,0.,1.));
#5306=DIRECTION('center_axis',(0.,0.,-1.));
#5307=DIRECTION('ref_axis',(1.,0.,0.));
#5308=DIRECTION('center_axis',(0.,0.,1.));
#5309=DIRECTION('ref_axis',(1.,0.,0.));
#5310=DIRECTION('center_axis',(0.,0.,1.));
#5311=DIRECTION('ref_axis',(1.,0.,0.));
#5312=DIRECTION('center_axis',(0.,0.,1.));
#5313=DIRECTION('ref_axis',(1.,0.,0.));
#5314=DIRECTION('center_axis',(0.,0.,1.));
#5315=DIRECTION('ref_axis',(1.,0.,0.));
#5316=DIRECTION('',(0.,0.,1.));
#5317=DIRECTION('center_axis',(0.,0.,-1.));
#5318=DIRECTION('ref_axis',(1.,0.,0.));
#5319=DIRECTION('center_axis',(0.,0.,1.));
#5320=DIRECTION('ref_axis',(1.,0.,0.));
#5321=DIRECTION('center_axis',(0.,0.,1.));
#5322=DIRECTION('ref_axis',(1.,0.,0.));
#5323=DIRECTION('center_axis',(0.,0.,1.));
#5324=DIRECTION('ref_axis',(1.,0.,0.));
#5325=DIRECTION('center_axis',(0.,0.,1.));
#5326=DIRECTION('ref_axis',(1.,0.,0.));
#5327=DIRECTION('',(0.,0.,1.));
#5328=DIRECTION('center_axis',(0.,0.,1.));
#5329=DIRECTION('ref_axis',(1.,0.,0.));
#5330=DIRECTION('center_axis',(0.,0.,1.));
#5331=DIRECTION('ref_axis',(1.,0.,0.));
#5332=DIRECTION('',(0.,0.,1.));
#5333=DIRECTION('center_axis',(0.,1.,0.));
#5334=DIRECTION('ref_axis',(-1.,0.,0.));
#5335=DIRECTION('',(-1.,0.,0.));
#5336=DIRECTION('',(0.,0.,1.));
#5337=DIRECTION('',(-1.,0.,0.));
#5338=DIRECTION('',(0.,0.,1.));
#5339=DIRECTION('center_axis',(1.,0.,0.));
#5340=DIRECTION('ref_axis',(0.,1.,0.));
#5341=DIRECTION('',(0.,1.,0.));
#5342=DIRECTION('',(0.,1.,0.));
#5343=DIRECTION('',(0.,0.,1.));
#5344=DIRECTION('center_axis',(0.,-1.,0.));
#5345=DIRECTION('ref_axis',(1.,0.,0.));
#5346=DIRECTION('',(1.,0.,0.));
#5347=DIRECTION('',(1.,0.,0.));
#5348=DIRECTION('',(0.,0.,1.));
#5349=DIRECTION('center_axis',(-1.,0.,0.));
#5350=DIRECTION('ref_axis',(0.,-1.,0.));
#5351=DIRECTION('',(0.,-1.,0.));
#5352=DIRECTION('',(0.,-1.,0.));
#5353=DIRECTION('center_axis',(0.,0.,1.));
#5354=DIRECTION('ref_axis',(1.,0.,0.));
#5355=DIRECTION('center_axis',(0.,0.,1.));
#5356=DIRECTION('ref_axis',(1.,0.,0.));
#6526=CARTESIAN_POINT('',(0.,0.,0.));
#6527=CARTESIAN_POINT('Origin',(3.,0.1,23.));
#6528=CARTESIAN_POINT('',(3.28284271247462,0.1,23.2828427124746));
#6529=CARTESIAN_POINT('',(2.71715728752538,0.1,23.2828427124746));
#6530=CARTESIAN_POINT('',(-5.1,0.1,23.2828427124746));
#6531=CARTESIAN_POINT('Origin',(3.,0.1,23.));
#6532=CARTESIAN_POINT('Origin',(3.,-2.1,23.));
#6533=CARTESIAN_POINT('',(2.6,-1.,23.));
#6534=CARTESIAN_POINT('Origin',(3.,-1.,23.));
#6535=CARTESIAN_POINT('',(2.6,-0.300000000000001,23.));
#6536=CARTESIAN_POINT('',(2.6,-2.1,23.));
#6537=CARTESIAN_POINT('',(2.73542486889354,-2.01044254631871E-17,23.3));
#6538=CARTESIAN_POINT('Ctrl Pts',(2.73542486889354,7.63278329429795E-17,
23.3));
#6539=CARTESIAN_POINT('Ctrl Pts',(2.73542486889354,-0.0201446772150695,
23.3));
#6540=CARTESIAN_POINT('Ctrl Pts',(2.73305334341681,-0.0403635841555968,
23.2979507721165));
#6541=CARTESIAN_POINT('Ctrl Pts',(2.7243365294397,-0.0797436599168342,23.2899048648568));
#6542=CARTESIAN_POINT('Ctrl Pts',(2.71802972961529,-0.0989142979472494,
23.2839128832536));
#6543=CARTESIAN_POINT('Ctrl Pts',(2.69593643019745,-0.153499080170581,23.2607687447172));
#6544=CARTESIAN_POINT('Ctrl Pts',(2.67718134717306,-0.186078125959879,23.2381859427521));
#6545=CARTESIAN_POINT('Ctrl Pts',(2.64492844776862,-0.237637949853887,23.186626118858));
#6546=CARTESIAN_POINT('Ctrl Pts',(2.62882756515854,-0.260548600882861,23.1539823555528));
#6547=CARTESIAN_POINT('Ctrl Pts',(2.60628603952013,-0.291765800294272,23.0804292530598));
#6548=CARTESIAN_POINT('Ctrl Pts',(2.6,-0.300000000000001,23.0394419468257));
#6549=CARTESIAN_POINT('Ctrl Pts',(2.6,-0.300000000000001,23.));
#6550=CARTESIAN_POINT('Ctrl Pts',(2.71715728752538,0.0999999999999983,23.2828427124746));
#6551=CARTESIAN_POINT('Ctrl Pts',(2.72174110582733,0.0870350039798468,23.2874265307766));
#6552=CARTESIAN_POINT('Ctrl Pts',(2.72568156083597,0.0736671922504066,23.2911463732685));
#6553=CARTESIAN_POINT('Ctrl Pts',(2.73305334341681,0.0403635841555971,23.2979507721165));
#6554=CARTESIAN_POINT('Ctrl Pts',(2.73542486889354,0.0201446772150696,23.3));
#6555=CARTESIAN_POINT('Ctrl Pts',(2.73542486889354,-6.93889390390723E-18,
23.3));
#6556=CARTESIAN_POINT('',(3.26457513110646,-1.40328932972683E-17,23.3));
#6557=CARTESIAN_POINT('Ctrl Pts',(3.26457513110646,-5.20417042793042E-18,
23.3));
#6558=CARTESIAN_POINT('Ctrl Pts',(3.26457513110646,0.0201446772150696,23.3));
#6559=CARTESIAN_POINT('Ctrl Pts',(3.26694665658319,0.0403635841555968,23.2979507721165));
#6560=CARTESIAN_POINT('Ctrl Pts',(3.27431843921387,0.0736671924755579,23.2911463732225));
#6561=CARTESIAN_POINT('Ctrl Pts',(3.27825889407742,0.0870350037104556,23.2874265308718));
#6562=CARTESIAN_POINT('Ctrl Pts',(3.28284271247462,0.0999999999999993,23.2828427124746));
#6563=CARTESIAN_POINT('',(3.28284271247462,0.1,22.7171572875254));
#6564=CARTESIAN_POINT('Ctrl Pts',(3.28284271247462,0.1,22.7171572875254));
#6565=CARTESIAN_POINT('Ctrl Pts',(3.27825889417267,0.0870350039798476,22.7125734692234));
#6566=CARTESIAN_POINT('Ctrl Pts',(3.27431843916403,0.0736671922504055,22.7088536267315));
#6567=CARTESIAN_POINT('Ctrl Pts',(3.26694665658319,0.0403635841555954,22.7020492278835));
#6568=CARTESIAN_POINT('Ctrl Pts',(3.26457513110646,0.0201446772150696,22.7));
#6569=CARTESIAN_POINT('Ctrl Pts',(3.26457513110646,0.,22.7));
#6570=CARTESIAN_POINT('Ctrl Pts',(3.26457513110646,-0.0201446772150696,
22.7));
#6571=CARTESIAN_POINT('Ctrl Pts',(3.26694665658319,-0.0403635841555971,
22.7020492278835));
#6572=CARTESIAN_POINT('Ctrl Pts',(3.2756634705603,-0.0797436599168345,22.7100951351432));
#6573=CARTESIAN_POINT('Ctrl Pts',(3.28197027038471,-0.0989142979472495,
22.7160871167464));
#6574=CARTESIAN_POINT('Ctrl Pts',(3.30406356980255,-0.153499080170581,22.7392312552828));
#6575=CARTESIAN_POINT('Ctrl Pts',(3.32281865282694,-0.186078125959879,22.7618140572479));
#6576=CARTESIAN_POINT('Ctrl Pts',(3.35507155223138,-0.237637949853888,22.813373881142));
#6577=CARTESIAN_POINT('Ctrl Pts',(3.37117243484146,-0.260548600882862,22.8460176444472));
#6578=CARTESIAN_POINT('Ctrl Pts',(3.39371396047987,-0.291765800294272,22.9195707469402));
#6579=CARTESIAN_POINT('Ctrl Pts',(3.4,-0.300000000000001,22.9605580531743));
#6580=CARTESIAN_POINT('Ctrl Pts',(3.4,-0.300000000000001,23.0394419468257));
#6581=CARTESIAN_POINT('Ctrl Pts',(3.39371396047987,-0.291765800294272,23.0804292530598));
#6582=CARTESIAN_POINT('Ctrl Pts',(3.37117243484146,-0.260548600882861,23.1539823555528));
#6583=CARTESIAN_POINT('Ctrl Pts',(3.35507155223138,-0.237637949853888,23.186626118858));
#6584=CARTESIAN_POINT('Ctrl Pts',(3.32281865282694,-0.186078125959879,23.2381859427521));
#6585=CARTESIAN_POINT('Ctrl Pts',(3.30406356980255,-0.153499080170581,23.2607687447172));
#6586=CARTESIAN_POINT('Ctrl Pts',(3.28197027038471,-0.0989142979472494,
23.2839128832536));
#6587=CARTESIAN_POINT('Ctrl Pts',(3.2756634705603,-0.0797436599168341,23.2899048648568));
#6588=CARTESIAN_POINT('Ctrl Pts',(3.26694665658319,-0.0403635841555968,
23.2979507721165));
#6589=CARTESIAN_POINT('Ctrl Pts',(3.26457513110646,-0.0201446772150696,
23.3));
#6590=CARTESIAN_POINT('Ctrl Pts',(3.26457513110646,2.08166817117217E-17,
23.3));
#6591=CARTESIAN_POINT('',(2.71715728752538,0.1,22.7171572875254));
#6592=CARTESIAN_POINT('Origin',(3.,0.1,23.));
#6593=CARTESIAN_POINT('Ctrl Pts',(2.6,-0.300000000000001,23.));
#6594=CARTESIAN_POINT('Ctrl Pts',(2.6,-0.300000000000001,22.9605580531743));
#6595=CARTESIAN_POINT('Ctrl Pts',(2.60628603952013,-0.291765800294272,22.9195707469402));
#6596=CARTESIAN_POINT('Ctrl Pts',(2.62882756515854,-0.260548600882862,22.8460176444472));
#6597=CARTESIAN_POINT('Ctrl Pts',(2.64492844776862,-0.237637949853888,22.813373881142));
#6598=CARTESIAN_POINT('Ctrl Pts',(2.67718134717306,-0.186078125959879,22.7618140572479));
#6599=CARTESIAN_POINT('Ctrl Pts',(2.69593643019745,-0.153499080170581,22.7392312552828));
#6600=CARTESIAN_POINT('Ctrl Pts',(2.71802972961529,-0.0989142979472494,
22.7160871167464));
#6601=CARTESIAN_POINT('Ctrl Pts',(2.7243365294397,-0.079743659916833,22.7100951351432));
#6602=CARTESIAN_POINT('Ctrl Pts',(2.73305334341681,-0.0403635841555955,
22.7020492278835));
#6603=CARTESIAN_POINT('Ctrl Pts',(2.73542486889354,-0.0201446772150696,
22.7));
#6604=CARTESIAN_POINT('Ctrl Pts',(2.73542486889354,0.,22.7));
#6605=CARTESIAN_POINT('Ctrl Pts',(2.73542486889354,0.0201446772150696,22.7));
#6606=CARTESIAN_POINT('Ctrl Pts',(2.73305334341681,0.0403635841555971,22.7020492278835));
#6607=CARTESIAN_POINT('Ctrl Pts',(2.72568156078613,0.0736671924755587,22.7088536267775));
#6608=CARTESIAN_POINT('Ctrl Pts',(2.72174110592258,0.0870350037104566,22.7125734691282));
#6609=CARTESIAN_POINT('Ctrl Pts',(2.71715728752538,0.0999999999999998,22.7171572875254));
#6610=CARTESIAN_POINT('Origin',(3.,0.1,23.));
#6611=CARTESIAN_POINT('',(-5.1,0.1,22.7171572875254));
#6612=CARTESIAN_POINT('Origin',(3.,-1.6,23.));
#6613=CARTESIAN_POINT('',(1.8,-1.5,23.));
#6614=CARTESIAN_POINT('Origin',(3.,-1.5,23.));
#6615=CARTESIAN_POINT('',(1.8,-1.,23.));
#6616=CARTESIAN_POINT('',(1.8,-1.6,23.));
#6617=CARTESIAN_POINT('Origin',(3.,-1.,23.));
#6618=CARTESIAN_POINT('Origin',(3.,-1.,23.));
#6619=CARTESIAN_POINT('Origin',(0.,0.1,23.));
#6620=CARTESIAN_POINT('',(0.282842712474617,0.1,23.2828427124746));
#6621=CARTESIAN_POINT('',(-0.282842712474617,0.1,23.2828427124746));
#6622=CARTESIAN_POINT('',(-5.1,0.1,23.2828427124746));
#6623=CARTESIAN_POINT('Origin',(0.,0.1,23.));
#6624=CARTESIAN_POINT('Origin',(0.,-2.1,23.));
#6625=CARTESIAN_POINT('',(-0.4,-1.,23.));
#6626=CARTESIAN_POINT('Origin',(0.,-1.,23.));
#6627=CARTESIAN_POINT('',(-0.4,-0.300000000000001,23.));
#6628=CARTESIAN_POINT('',(-0.4,-2.1,23.));
#6629=CARTESIAN_POINT('',(-0.264575131106458,-4.49191417939589E-18,23.3));
#6630=CARTESIAN_POINT('Ctrl Pts',(-0.264575131106458,1.04083408558608E-16,
23.3));
#6631=CARTESIAN_POINT('Ctrl Pts',(-0.264575131106458,-0.0201446772150695,
23.3));
#6632=CARTESIAN_POINT('Ctrl Pts',(-0.266946656583192,-0.0403635841555969,
23.2979507721165));
#6633=CARTESIAN_POINT('Ctrl Pts',(-0.275663470560296,-0.0797436599168343,
23.2899048648568));
#6634=CARTESIAN_POINT('Ctrl Pts',(-0.281970270384707,-0.0989142979472496,
23.2839128832536));
#6635=CARTESIAN_POINT('Ctrl Pts',(-0.30406356980255,-0.153499080170581,
23.2607687447172));
#6636=CARTESIAN_POINT('Ctrl Pts',(-0.322818652826944,-0.186078125959879,
23.2381859427521));
#6637=CARTESIAN_POINT('Ctrl Pts',(-0.35507155223138,-0.237637949853888,
23.186626118858));
#6638=CARTESIAN_POINT('Ctrl Pts',(-0.371172434841458,-0.260548600882862,
23.1539823555528));
#6639=CARTESIAN_POINT('Ctrl Pts',(-0.393713960479866,-0.291765800294272,
23.0804292530598));
#6640=CARTESIAN_POINT('Ctrl Pts',(-0.4,-0.300000000000001,23.0394419468257));
#6641=CARTESIAN_POINT('Ctrl Pts',(-0.4,-0.300000000000001,23.));
#6642=CARTESIAN_POINT('Ctrl Pts',(-0.282842712474619,0.099999999999999,
23.2828427124746));
#6643=CARTESIAN_POINT('Ctrl Pts',(-0.278258894172666,0.087035003979848,
23.2874265307766));
#6644=CARTESIAN_POINT('Ctrl Pts',(-0.274318439164031,0.0736671922504069,
23.2911463732685));
#6645=CARTESIAN_POINT('Ctrl Pts',(-0.266946656583192,0.0403635841555971,
23.2979507721165));
#6646=CARTESIAN_POINT('Ctrl Pts',(-0.264575131106458,0.0201446772150696,
23.3));
#6647=CARTESIAN_POINT('Ctrl Pts',(-0.264575131106458,-2.08166817117217E-17,
23.3));
#6648=CARTESIAN_POINT('',(0.264575131106458,1.11205971043954E-17,23.3));
#6649=CARTESIAN_POINT('Ctrl Pts',(0.264575131106458,-7.63278329429795E-17,
23.3));
#6650=CARTESIAN_POINT('Ctrl Pts',(0.264575131106458,0.0201446772150695,
23.3));
#6651=CARTESIAN_POINT('Ctrl Pts',(0.266946656583192,0.0403635841555971,
23.2979507721165));
#6652=CARTESIAN_POINT('Ctrl Pts',(0.274318439213869,0.0736671924755586,
23.2911463732225));
#6653=CARTESIAN_POINT('Ctrl Pts',(0.278258894077421,0.0870350037104561,
23.2874265308718));
#6654=CARTESIAN_POINT('Ctrl Pts',(0.282842712474618,0.0999999999999992,
23.2828427124746));
#6655=CARTESIAN_POINT('',(0.282842712474617,0.1,22.7171572875254));
#6656=CARTESIAN_POINT('Ctrl Pts',(0.282842712474619,0.1,22.7171572875254));
#6657=CARTESIAN_POINT('Ctrl Pts',(0.278258894172666,0.0870350039798482,
22.7125734692234));
#6658=CARTESIAN_POINT('Ctrl Pts',(0.274318439164031,0.0736671922504066,
22.7088536267315));
#6659=CARTESIAN_POINT('Ctrl Pts',(0.266946656583192,0.0403635841555971,
22.7020492278835));
#6660=CARTESIAN_POINT('Ctrl Pts',(0.264575131106458,0.0201446772150696,
22.7));
#6661=CARTESIAN_POINT('Ctrl Pts',(0.264575131106458,0.,22.7));
#6662=CARTESIAN_POINT('Ctrl Pts',(0.264575131106458,-0.0201446772150696,
22.7));
#6663=CARTESIAN_POINT('Ctrl Pts',(0.266946656583192,-0.0403635841555971,
22.7020492278835));
#6664=CARTESIAN_POINT('Ctrl Pts',(0.275663470560296,-0.0797436599168345,
22.7100951351432));
#6665=CARTESIAN_POINT('Ctrl Pts',(0.281970270384707,-0.0989142979472497,
22.7160871167464));
#6666=CARTESIAN_POINT('Ctrl Pts',(0.30406356980255,-0.153499080170581,22.7392312552828));
#6667=CARTESIAN_POINT('Ctrl Pts',(0.322818652826944,-0.186078125959879,
22.7618140572479));
#6668=CARTESIAN_POINT('Ctrl Pts',(0.35507155223138,-0.237637949853888,22.813373881142));
#6669=CARTESIAN_POINT('Ctrl Pts',(0.371172434841456,-0.260548600882859,
22.8460176444472));
#6670=CARTESIAN_POINT('Ctrl Pts',(0.393713960479865,-0.291765800294271,
22.9195707469402));
#6671=CARTESIAN_POINT('Ctrl Pts',(0.4,-0.300000000000001,22.9605580531743));
#6672=CARTESIAN_POINT('Ctrl Pts',(0.4,-0.300000000000001,23.0394419468257));
#6673=CARTESIAN_POINT('Ctrl Pts',(0.393713960479866,-0.291765800294272,
23.0804292530598));
#6674=CARTESIAN_POINT('Ctrl Pts',(0.371172434841458,-0.260548600882862,
23.1539823555528));
#6675=CARTESIAN_POINT('Ctrl Pts',(0.35507155223138,-0.237637949853888,23.186626118858));
#6676=CARTESIAN_POINT('Ctrl Pts',(0.322818652826944,-0.186078125959879,
23.2381859427521));
#6677=CARTESIAN_POINT('Ctrl Pts',(0.304063569802549,-0.153499080170581,
23.2607687447172));
#6678=CARTESIAN_POINT('Ctrl Pts',(0.281970270384707,-0.0989142979472497,
23.2839128832536));
#6679=CARTESIAN_POINT('Ctrl Pts',(0.275663470560296,-0.0797436599168345,
23.2899048648568));
#6680=CARTESIAN_POINT('Ctrl Pts',(0.266946656583192,-0.0403635841555971,
23.2979507721165));
#6681=CARTESIAN_POINT('Ctrl Pts',(0.264575131106458,-0.0201446772150695,
23.3));
#6682=CARTESIAN_POINT('Ctrl Pts',(0.264575131106458,8.67361737988404E-17,
23.3));
#6683=CARTESIAN_POINT('',(-0.282842712474617,0.1,22.7171572875254));
#6684=CARTESIAN_POINT('Origin',(0.,0.1,23.));
#6685=CARTESIAN_POINT('Ctrl Pts',(-0.4,-0.300000000000001,23.));
#6686=CARTESIAN_POINT('Ctrl Pts',(-0.4,-0.300000000000001,22.9605580531743));
#6687=CARTESIAN_POINT('Ctrl Pts',(-0.393713960479866,-0.291765800294272,
22.9195707469402));
#6688=CARTESIAN_POINT('Ctrl Pts',(-0.371172434841458,-0.260548600882862,
22.8460176444472));
#6689=CARTESIAN_POINT('Ctrl Pts',(-0.35507155223138,-0.237637949853888,
22.813373881142));
#6690=CARTESIAN_POINT('Ctrl Pts',(-0.322818652826944,-0.186078125959879,
22.7618140572479));
#6691=CARTESIAN_POINT('Ctrl Pts',(-0.30406356980255,-0.153499080170581,
22.7392312552828));
#6692=CARTESIAN_POINT('Ctrl Pts',(-0.281970270384707,-0.0989142979472497,
22.7160871167464));
#6693=CARTESIAN_POINT('Ctrl Pts',(-0.275663470560296,-0.0797436599168337,
22.7100951351432));
#6694=CARTESIAN_POINT('Ctrl Pts',(-0.266946656583192,-0.0403635841555955,
22.7020492278835));
#6695=CARTESIAN_POINT('Ctrl Pts',(-0.264575131106458,-0.0201446772150697,
22.7));
#6696=CARTESIAN_POINT('Ctrl Pts',(-0.264575131106458,0.,22.7));
#6697=CARTESIAN_POINT('Ctrl Pts',(-0.264575131106458,0.0201446772150696,
22.7));
#6698=CARTESIAN_POINT('Ctrl Pts',(-0.266946656583192,0.0403635841555971,
22.7020492278835));
#6699=CARTESIAN_POINT('Ctrl Pts',(-0.274318439213869,0.0736671924755591,
22.7088536267775));
#6700=CARTESIAN_POINT('Ctrl Pts',(-0.27825889407742,0.087035003710456,22.7125734691282));
#6701=CARTESIAN_POINT('Ctrl Pts',(-0.282842712474618,0.0999999999999995,
22.7171572875254));
#6702=CARTESIAN_POINT('Origin',(0.,0.1,23.));
#6703=CARTESIAN_POINT('',(-5.1,0.1,22.7171572875254));
#6704=CARTESIAN_POINT('Origin',(0.,-1.6,23.));
#6705=CARTESIAN_POINT('',(-1.2,-1.5,23.));
#6706=CARTESIAN_POINT('Origin',(0.,-1.5,23.));
#6707=CARTESIAN_POINT('',(-1.2,-1.,23.));
#6708=CARTESIAN_POINT('',(-1.2,-1.6,23.));
#6709=CARTESIAN_POINT('Origin',(0.,-1.,23.));
#6710=CARTESIAN_POINT('Origin',(0.,-1.,23.));
#6711=CARTESIAN_POINT('Origin',(-3.,0.1,23.));
#6712=CARTESIAN_POINT('',(-2.71715728752538,0.1,23.2828427124746));
#6713=CARTESIAN_POINT('',(-3.28284271247462,0.1,23.2828427124746));
#6714=CARTESIAN_POINT('',(-5.1,0.1,23.2828427124746));
#6715=CARTESIAN_POINT('Origin',(-3.,0.1,23.));
#6716=CARTESIAN_POINT('Origin',(-3.,-2.1,23.));
#6717=CARTESIAN_POINT('',(-3.4,-1.,23.));
#6718=CARTESIAN_POINT('Origin',(-3.,-1.,23.));
#6719=CARTESIAN_POINT('',(-3.4,-0.300000000000001,23.));
#6720=CARTESIAN_POINT('',(-3.4,-2.1,23.));
#6721=CARTESIAN_POINT('',(-3.26457513110646,-2.75719070341908E-18,23.3));
#6722=CARTESIAN_POINT('Ctrl Pts',(-3.26457513110646,1.14491749414469E-16,
23.3));
#6723=CARTESIAN_POINT('Ctrl Pts',(-3.26457513110646,-0.0201446772150695,
23.3));
#6724=CARTESIAN_POINT('Ctrl Pts',(-3.26694665658319,-0.0403635841555969,
23.2979507721165));
#6725=CARTESIAN_POINT('Ctrl Pts',(-3.27566347056029,-0.0797436599168342,
23.2899048648568));
#6726=CARTESIAN_POINT('Ctrl Pts',(-3.28197027038471,-0.0989142979472495,
23.2839128832536));
#6727=CARTESIAN_POINT('Ctrl Pts',(-3.30406356980255,-0.153499080170581,
23.2607687447172));
#6728=CARTESIAN_POINT('Ctrl Pts',(-3.32281865282694,-0.186078125959879,
23.2381859427521));
#6729=CARTESIAN_POINT('Ctrl Pts',(-3.35507155223138,-0.237637949853887,
23.186626118858));
#6730=CARTESIAN_POINT('Ctrl Pts',(-3.37117243484146,-0.260548600882861,
23.1539823555528));
#6731=CARTESIAN_POINT('Ctrl Pts',(-3.39371396047987,-0.291765800294272,
23.0804292530598));
#6732=CARTESIAN_POINT('Ctrl Pts',(-3.4,-0.300000000000001,23.0394419468257));
#6733=CARTESIAN_POINT('Ctrl Pts',(-3.4,-0.300000000000001,23.));
#6734=CARTESIAN_POINT('Ctrl Pts',(-3.28284271247462,0.0999999999999976,
23.2828427124746));
#6735=CARTESIAN_POINT('Ctrl Pts',(-3.27825889417267,0.0870350039798463,
23.2874265307766));
#6736=CARTESIAN_POINT('Ctrl Pts',(-3.27431843916403,0.0736671922504077,
23.2911463732685));
#6737=CARTESIAN_POINT('Ctrl Pts',(-3.26694665658319,0.0403635841555971,
23.2979507721165));
#6738=CARTESIAN_POINT('Ctrl Pts',(-3.26457513110646,0.0201446772150696,
23.3));
#6739=CARTESIAN_POINT('Ctrl Pts',(-3.26457513110646,-1.38777878078145E-17,
23.3));
#6740=CARTESIAN_POINT('',(-2.73542486889354,8.57137065713981E-17,23.3));
#6741=CARTESIAN_POINT('Ctrl Pts',(-2.73542486889354,9.36750677027476E-17,
23.3));
#6742=CARTESIAN_POINT('Ctrl Pts',(-2.73542486889354,0.0201446772150697,
23.3));
#6743=CARTESIAN_POINT('Ctrl Pts',(-2.73305334341681,0.0403635841555968,
23.2979507721165));
#6744=CARTESIAN_POINT('Ctrl Pts',(-2.72568156078613,0.0736671924755579,
23.2911463732225));
#6745=CARTESIAN_POINT('Ctrl Pts',(-2.72174110592258,0.0870350037104556,
23.2874265308718));
#6746=CARTESIAN_POINT('Ctrl Pts',(-2.71715728752538,0.0999999999999993,
23.2828427124746));
#6747=CARTESIAN_POINT('',(-2.71715728752538,0.1,22.7171572875254));
#6748=CARTESIAN_POINT('Ctrl Pts',(-2.71715728752538,0.0999999999999998,
22.7171572875254));
#6749=CARTESIAN_POINT('Ctrl Pts',(-2.72174110582733,0.0870350039798475,
22.7125734692234));
#6750=CARTESIAN_POINT('Ctrl Pts',(-2.72568156083597,0.0736671922504053,
22.7088536267315));
#6751=CARTESIAN_POINT('Ctrl Pts',(-2.73305334341681,0.0403635841555956,
22.7020492278835));
#6752=CARTESIAN_POINT('Ctrl Pts',(-2.73542486889354,0.0201446772150696,
22.7));
#6753=CARTESIAN_POINT('Ctrl Pts',(-2.73542486889354,0.,22.7));
#6754=CARTESIAN_POINT('Ctrl Pts',(-2.73542486889354,-0.0201446772150696,
22.7));
#6755=CARTESIAN_POINT('Ctrl Pts',(-2.73305334341681,-0.0403635841555972,
22.7020492278835));
#6756=CARTESIAN_POINT('Ctrl Pts',(-2.72433652943971,-0.0797436599168346,
22.7100951351432));
#6757=CARTESIAN_POINT('Ctrl Pts',(-2.71802972961529,-0.0989142979472495,
22.7160871167464));
#6758=CARTESIAN_POINT('Ctrl Pts',(-2.69593643019745,-0.153499080170581,
22.7392312552828));
#6759=CARTESIAN_POINT('Ctrl Pts',(-2.67718134717306,-0.186078125959879,
22.7618140572479));
#6760=CARTESIAN_POINT('Ctrl Pts',(-2.64492844776862,-0.237637949853888,
22.813373881142));
#6761=CARTESIAN_POINT('Ctrl Pts',(-2.62882756515854,-0.260548600882862,
22.8460176444472));
#6762=CARTESIAN_POINT('Ctrl Pts',(-2.60628603952013,-0.291765800294272,
22.9195707469402));
#6763=CARTESIAN_POINT('Ctrl Pts',(-2.6,-0.300000000000001,22.9605580531743));
#6764=CARTESIAN_POINT('Ctrl Pts',(-2.6,-0.300000000000001,23.0394419468257));
#6765=CARTESIAN_POINT('Ctrl Pts',(-2.60628603952013,-0.291765800294272,
23.0804292530598));
#6766=CARTESIAN_POINT('Ctrl Pts',(-2.62882756515854,-0.260548600882861,
23.1539823555528));
#6767=CARTESIAN_POINT('Ctrl Pts',(-2.64492844776862,-0.237637949853888,
23.186626118858));
#6768=CARTESIAN_POINT('Ctrl Pts',(-2.67718134717306,-0.186078125959879,
23.2381859427521));
#6769=CARTESIAN_POINT('Ctrl Pts',(-2.69593643019745,-0.153499080170581,
23.2607687447172));
#6770=CARTESIAN_POINT('Ctrl Pts',(-2.71802972961529,-0.0989142979472495,
23.2839128832536));
#6771=CARTESIAN_POINT('Ctrl Pts',(-2.72433652943971,-0.0797436599168343,
23.2899048648568));
#6772=CARTESIAN_POINT('Ctrl Pts',(-2.73305334341681,-0.0403635841555968,
23.2979507721165));
#6773=CARTESIAN_POINT('Ctrl Pts',(-2.73542486889354,-0.0201446772150696,
23.3));
#6774=CARTESIAN_POINT('Ctrl Pts',(-2.73542486889354,3.29597460435593E-17,
23.3));
#6775=CARTESIAN_POINT('',(-3.28284271247462,0.1,22.7171572875254));
#6776=CARTESIAN_POINT('Origin',(-3.,0.1,23.));
#6777=CARTESIAN_POINT('Ctrl Pts',(-3.4,-0.300000000000001,23.));
#6778=CARTESIAN_POINT('Ctrl Pts',(-3.4,-0.300000000000001,22.9605580531743));
#6779=CARTESIAN_POINT('Ctrl Pts',(-3.39371396047987,-0.291765800294272,
22.9195707469402));
#6780=CARTESIAN_POINT('Ctrl Pts',(-3.37117243484146,-0.260548600882862,
22.8460176444472));
#6781=CARTESIAN_POINT('Ctrl Pts',(-3.35507155223138,-0.237637949853888,
22.813373881142));
#6782=CARTESIAN_POINT('Ctrl Pts',(-3.32281865282694,-0.186078125959879,
22.7618140572479));
#6783=CARTESIAN_POINT('Ctrl Pts',(-3.30406356980255,-0.153499080170581,
22.7392312552828));
#6784=CARTESIAN_POINT('Ctrl Pts',(-3.28197027038471,-0.0989142979472495,
22.7160871167464));
#6785=CARTESIAN_POINT('Ctrl Pts',(-3.27566347056029,-0.0797436599168329,
22.7100951351432));
#6786=CARTESIAN_POINT('Ctrl Pts',(-3.26694665658319,-0.0403635841555953,
22.7020492278835));
#6787=CARTESIAN_POINT('Ctrl Pts',(-3.26457513110646,-0.0201446772150696,
22.7));
#6788=CARTESIAN_POINT('Ctrl Pts',(-3.26457513110646,0.,22.7));
#6789=CARTESIAN_POINT('Ctrl Pts',(-3.26457513110646,0.0201446772150696,
22.7));
#6790=CARTESIAN_POINT('Ctrl Pts',(-3.26694665658319,0.0403635841555971,
22.7020492278835));
#6791=CARTESIAN_POINT('Ctrl Pts',(-3.27431843921387,0.0736671924755593,
22.7088536267775));
#6792=CARTESIAN_POINT('Ctrl Pts',(-3.27825889407742,0.0870350037104561,
22.7125734691282));
#6793=CARTESIAN_POINT('Ctrl Pts',(-3.28284271247462,0.0999999999999997,
22.7171572875254));
#6794=CARTESIAN_POINT('Origin',(-3.,0.1,23.));
#6795=CARTESIAN_POINT('',(-5.1,0.1,22.7171572875254));
#6796=CARTESIAN_POINT('Origin',(-3.,-1.6,23.));
#6797=CARTESIAN_POINT('',(-4.2,-1.5,23.));
#6798=CARTESIAN_POINT('Origin',(-3.,-1.5,23.));
#6799=CARTESIAN_POINT('',(-4.2,-1.,23.));
#6800=CARTESIAN_POINT('',(-4.2,-1.6,23.));
#6801=CARTESIAN_POINT('Origin',(-3.,-1.,23.));
#6802=CARTESIAN_POINT('Origin',(-3.,-1.,23.));
#6803=CARTESIAN_POINT('Origin',(3.6,0.,23.));
#6804=CARTESIAN_POINT('',(3.6,-8.38883057415935E-17,23.685));
#6805=CARTESIAN_POINT('Origin',(3.6,0.,23.));
#6806=CARTESIAN_POINT('',(5.,8.38883057415935E-17,23.685));
#6807=CARTESIAN_POINT('',(3.6,-8.38883057415935E-17,23.685));
#6808=CARTESIAN_POINT('Origin',(5.,0.,23.));
#6809=CARTESIAN_POINT('',(4.3,0.6,23.3304920573932));
#6810=CARTESIAN_POINT('Ctrl Pts',(4.3,0.6,23.3304920573932));
#6811=CARTESIAN_POINT('Ctrl Pts',(4.27077753133383,0.6,23.3304920573932));
#6812=CARTESIAN_POINT('Ctrl Pts',(4.24011034888269,0.603494484869573,23.3243525399112));
#6813=CARTESIAN_POINT('Ctrl Pts',(4.18479795469579,0.615901327435478,23.3001263251791));
#6814=CARTESIAN_POINT('Ctrl Pts',(4.16014428890256,0.624655274357919,23.2819781026066));
#6815=CARTESIAN_POINT('Ctrl Pts',(4.12028928729214,0.641942325510241,23.2401640721199));
#6816=CARTESIAN_POINT('Ctrl Pts',(4.10113513579261,0.652637676126791,23.2100112664292));
#6817=CARTESIAN_POINT('Ctrl Pts',(4.07712932095812,0.667553927651758,23.1560425561636));
#6818=CARTESIAN_POINT('Ctrl Pts',(4.06787168700093,0.674162120990136,23.1254789195617));
#6819=CARTESIAN_POINT('Ctrl Pts',(4.05607440793796,0.682897228967308,23.0623771974352));
#6820=CARTESIAN_POINT('Ctrl Pts',(4.05347413928758,0.684999999999999,23.0298471208273));
#6821=CARTESIAN_POINT('Ctrl Pts',(4.05347413928758,0.684999999999999,22.9701528791727));
#6822=CARTESIAN_POINT('Ctrl Pts',(4.05607440793796,0.682897228967308,22.9376228025648));
#6823=CARTESIAN_POINT('Ctrl Pts',(4.06787168700092,0.674162120990137,22.8745210804384));
#6824=CARTESIAN_POINT('Ctrl Pts',(4.07712932095812,0.667553927651758,22.8439574438364));
#6825=CARTESIAN_POINT('Ctrl Pts',(4.10113513579261,0.652637676126791,22.7899887335708));
#6826=CARTESIAN_POINT('Ctrl Pts',(4.12028928729214,0.641942325510241,22.7598359278801));
#6827=CARTESIAN_POINT('Ctrl Pts',(4.16014428890256,0.624655274357919,22.7180218973934));
#6828=CARTESIAN_POINT('Ctrl Pts',(4.18479795469579,0.615901327435478,22.6998736748209));
#6829=CARTESIAN_POINT('Ctrl Pts',(4.24011034888269,0.603494484869573,22.6756474600888));
#6830=CARTESIAN_POINT('Ctrl Pts',(4.27077753133383,0.6,22.6695079426068));
#6831=CARTESIAN_POINT('Ctrl Pts',(4.32922246866617,0.6,22.6695079426068));
#6832=CARTESIAN_POINT('Ctrl Pts',(4.3598896511173,0.603494484869573,22.6756474600888));
#6833=CARTESIAN_POINT('Ctrl Pts',(4.41520204530421,0.615901327435478,22.6998736748209));
#6834=CARTESIAN_POINT('Ctrl Pts',(4.43985571109744,0.624655274357919,22.7180218973934));
#6835=CARTESIAN_POINT('Ctrl Pts',(4.47971071270786,0.641942325510241,22.7598359278801));
#6836=CARTESIAN_POINT('Ctrl Pts',(4.49886486420739,0.652637676126791,22.7899887335708));
#6837=CARTESIAN_POINT('Ctrl Pts',(4.52287067904188,0.667553927651758,22.8439574438364));
#6838=CARTESIAN_POINT('Ctrl Pts',(4.53212831299907,0.674162120990137,22.8745210804384));
#6839=CARTESIAN_POINT('Ctrl Pts',(4.54392559206204,0.682897228967308,22.9376228025648));
#6840=CARTESIAN_POINT('Ctrl Pts',(4.54652586071242,0.684999999999999,22.9701528791727));
#6841=CARTESIAN_POINT('Ctrl Pts',(4.54652586071242,0.684999999999999,23.0298471208273));
#6842=CARTESIAN_POINT('Ctrl Pts',(4.54392559206204,0.682897228967308,23.0623771974352));
#6843=CARTESIAN_POINT('Ctrl Pts',(4.53212831299907,0.674162120990136,23.1254789195617));
#6844=CARTESIAN_POINT('Ctrl Pts',(4.52287067904188,0.667553927651758,23.1560425561636));
#6845=CARTESIAN_POINT('Ctrl Pts',(4.49886486420739,0.652637676126791,23.2100112664292));
#6846=CARTESIAN_POINT('Ctrl Pts',(4.47971071270786,0.641942325510241,23.2401640721199));
#6847=CARTESIAN_POINT('Ctrl Pts',(4.43985571109744,0.624655274357919,23.2819781026066));
#6848=CARTESIAN_POINT('Ctrl Pts',(4.41520204530421,0.615901327435478,23.3001263251791));
#6849=CARTESIAN_POINT('Ctrl Pts',(4.3598896511173,0.603494484869573,23.3243525399112));
#6850=CARTESIAN_POINT('Ctrl Pts',(4.32922246866617,0.6,23.3304920573932));
#6851=CARTESIAN_POINT('Ctrl Pts',(4.3,0.6,23.3304920573932));
#6852=CARTESIAN_POINT('Origin',(3.6,0.,23.));
#6853=CARTESIAN_POINT('',(3.6,-3.67394039744207E-17,23.3));
#6854=CARTESIAN_POINT('Origin',(3.6,0.,23.));
#6855=CARTESIAN_POINT('Origin',(-5.1,0.,23.));
#6856=CARTESIAN_POINT('',(-5.,-3.67394039744207E-17,23.3));
#6857=CARTESIAN_POINT('Origin',(-5.,0.,23.));
#6858=CARTESIAN_POINT('',(-5.1,-3.67394039744207E-17,23.3));
#6859=CARTESIAN_POINT('',(-5.1,-3.67394039744207E-17,23.3));
#6860=CARTESIAN_POINT('',(-5.1,-3.67394039744207E-17,23.3));
#6861=CARTESIAN_POINT('',(-5.1,-3.67394039744207E-17,23.3));
#6862=CARTESIAN_POINT('Origin',(-4.3,1.,22.3));
#6863=CARTESIAN_POINT('',(-4.7,1.,22.3));
#6864=CARTESIAN_POINT('Origin',(-4.3,1.,22.3));
#6865=CARTESIAN_POINT('',(-4.7,1.,24.5));
#6866=CARTESIAN_POINT('',(-4.7,1.,22.3));
#6867=CARTESIAN_POINT('Origin',(-4.3,1.,24.5));
#6868=CARTESIAN_POINT('Origin',(-4.3,1.,22.3));
#6869=CARTESIAN_POINT('',(-4.525,1.,22.3));
#6870=CARTESIAN_POINT('Origin',(-4.3,1.,22.3));
#6871=CARTESIAN_POINT('Origin',(4.3,1.,22.3));
#6872=CARTESIAN_POINT('',(3.9,1.,22.3));
#6873=CARTESIAN_POINT('Origin',(4.3,1.,22.3));
#6874=CARTESIAN_POINT('',(3.9,1.,24.5));
#6875=CARTESIAN_POINT('',(3.9,1.,22.3));
#6876=CARTESIAN_POINT('Origin',(4.3,1.,24.5));
#6877=CARTESIAN_POINT('Origin',(4.3,1.,22.3));
#6878=CARTESIAN_POINT('',(4.075,1.,22.3));
#6879=CARTESIAN_POINT('Origin',(4.3,1.,22.3));
#6880=CARTESIAN_POINT('Origin',(-4.3,1.,21.4));
#6881=CARTESIAN_POINT('',(-4.525,1.,21.5));
#6882=CARTESIAN_POINT('Origin',(-4.3,1.,21.5));
#6883=CARTESIAN_POINT('',(-4.525,1.,21.4));
#6884=CARTESIAN_POINT('Origin',(4.3,1.,21.4));
#6885=CARTESIAN_POINT('',(4.075,1.,21.5));
#6886=CARTESIAN_POINT('Origin',(4.3,1.,21.5));
#6887=CARTESIAN_POINT('',(4.075,1.,21.4));
#6888=CARTESIAN_POINT('Origin',(5.,1.5,21.5));
#6889=CARTESIAN_POINT('',(5.,1.5,21.5));
#6890=CARTESIAN_POINT('',(-5.,1.5,21.5));
#6891=CARTESIAN_POINT('',(5.,1.5,21.5));
#6892=CARTESIAN_POINT('',(-5.,1.5,24.5));
#6893=CARTESIAN_POINT('',(-5.,1.5,21.5));
#6894=CARTESIAN_POINT('',(5.,1.5,24.5));
#6895=CARTESIAN_POINT('',(5.,1.5,24.5));
#6896=CARTESIAN_POINT('',(5.,1.5,21.5));
#6897=CARTESIAN_POINT('Origin',(5.,-1.5,21.5));
#6898=CARTESIAN_POINT('',(5.,-1.5,21.5));
#6899=CARTESIAN_POINT('',(5.,-1.5,21.5));
#6900=CARTESIAN_POINT('',(5.,-1.5,24.5));
#6901=CARTESIAN_POINT('',(5.,-1.5,24.5));
#6902=CARTESIAN_POINT('',(5.,-1.5,21.5));
#6903=CARTESIAN_POINT('Origin',(-5.,-1.5,21.5));
#6904=CARTESIAN_POINT('',(-5.,-1.5,21.5));
#6905=CARTESIAN_POINT('',(-5.,-1.5,21.5));
#6906=CARTESIAN_POINT('',(-5.,-1.5,24.5));
#6907=CARTESIAN_POINT('',(-5.,-1.5,24.5));
#6908=CARTESIAN_POINT('',(-5.,-1.5,21.5));
#6909=CARTESIAN_POINT('Origin',(-5.,1.5,21.5));
#6910=CARTESIAN_POINT('',(-5.,1.5,21.5));
#6911=CARTESIAN_POINT('',(-5.,1.5,24.5));
#6912=CARTESIAN_POINT('Origin',(0.,0.,24.5));
#6913=CARTESIAN_POINT('Origin',(0.,0.,21.5));
#7840=UNCERTAINTY_MEASURE_WITH_UNIT(LENGTH_MEASURE(0.001),#7898,
'DISTANCE_ACCURACY_VALUE',
'Maximum model space distance between geometric entities at asserted c
onnectivities');
#7865=UNCERTAINTY_MEASURE_WITH_UNIT(LENGTH_MEASURE(0.001),#7898,
'DISTANCE_ACCURACY_VALUE',
'Maximum model space distance between geometric entities at asserted c
onnectivities');
#7872=(
GEOMETRIC_REPRESENTATION_CONTEXT(3)
GLOBAL_UNCERTAINTY_ASSIGNED_CONTEXT((#7840))
GLOBAL_UNIT_ASSIGNED_CONTEXT((#7898,#7900,#7901))
REPRESENTATION_CONTEXT('','3D')
);
#7897=(
GEOMETRIC_REPRESENTATION_CONTEXT(3)
GLOBAL_UNCERTAINTY_ASSIGNED_CONTEXT((#7865))
GLOBAL_UNIT_ASSIGNED_CONTEXT((#7898,#7900,#7901))
REPRESENTATION_CONTEXT('','3D')
);
#7898=(
LENGTH_UNIT()
NAMED_UNIT(*)
SI_UNIT(.CENTI.,.METRE.)
);
#7900=(
NAMED_UNIT(*)
PLANE_ANGLE_UNIT()
SI_UNIT($,.RADIAN.)
);
#7901=(
NAMED_UNIT(*)
SI_UNIT($,.STERADIAN.)
SOLID_ANGLE_UNIT()
);
#7908=SHAPE_DEFINITION_REPRESENTATION(#7939,#8005);
#7939=PRODUCT_DEFINITION_SHAPE('',$,#8037);
#8005=SHAPE_REPRESENTATION('',(#4631),#7872);
#8030=PRODUCT_DEFINITION_CONTEXT('part definition',#8125,'design');
#8037=PRODUCT_DEFINITION('Manifold','Manifold',#8068,#8030);
#8068=PRODUCT_DEFINITION_FORMATION('',$,#8133);
#8125=APPLICATION_CONTEXT(
'Core Data for Automotive Mechanical Design Process');
#8126=PRODUCT_CONTEXT('part definition',#8125,'mechanical');
#8133=PRODUCT('Manifold','Manifold','Manifold',(#8126));
#8228=COLOUR_RGB('Off White',0.89,0.88,0.83);
#8229=FILL_AREA_STYLE_COLOUR('',#8228);
#8230=FILL_AREA_STYLE('',(#8229));
#8231=SURFACE_STYLE_FILL_AREA(#8230);
#8232=SURFACE_SIDE_STYLE('',(#8231));
#8233=SURFACE_STYLE_USAGE(.BOTH.,#8232);
#8234=PRESENTATION_STYLE_ASSIGNMENT((#8233));
ENDSEC;
END-ISO-10303-21;
